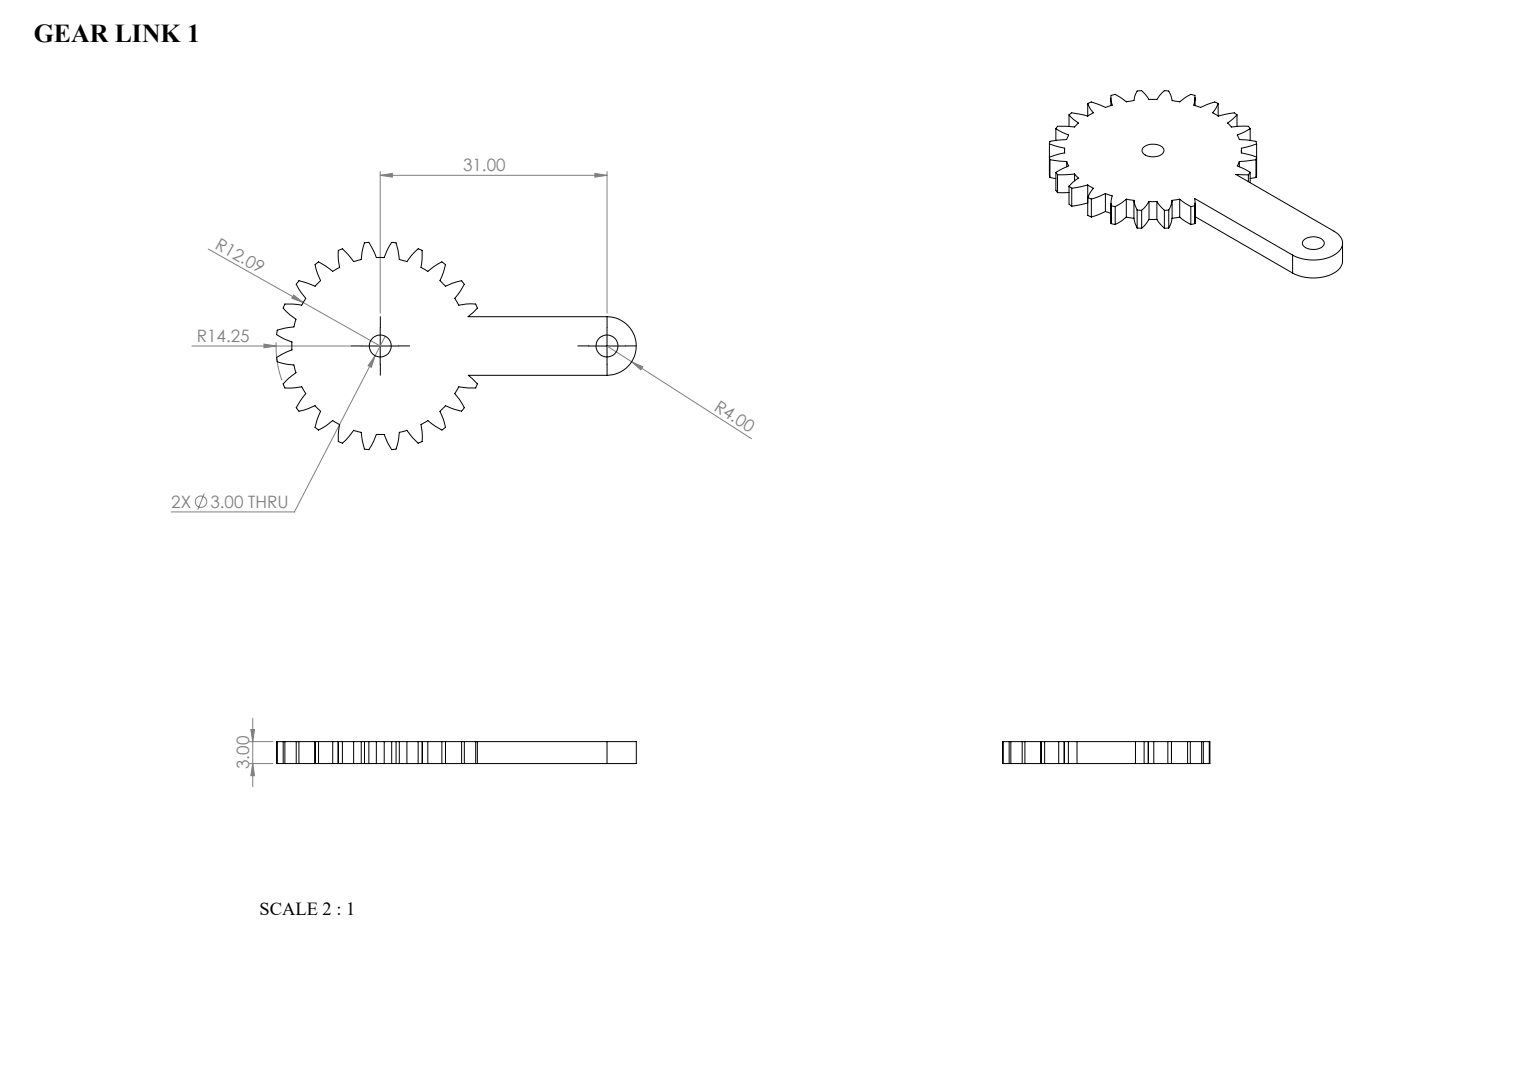
ISO-10303-21;
HEADER;
FILE_DESCRIPTION (('STEP AP214'),
    '1' );
FILE_NAME ('gear-link-1.step',
    '2026-10-11T23:18:24',
    ( '' ),
    ( '' ),
    'SwSTEP 2.0',
    'SolidWorks 2021',
    '' );
FILE_SCHEMA (( 'AUTOMOTIVE_DESIGN' ));
ENDSEC;

DATA;
#5=FACE_OUTER_BOUND ( 'NONE', #2599, .T. ) ;
#10=B_SPLINE_CURVE_WITH_KNOTS ( 'NONE', 3,
 ( #6640, #5405, #12919, #3466 ),
 .UNSPECIFIED., .F., .F.,
 ( 4, 4 ),
 ( 0.1547128134717859205, 1.000000000000000000 ),
 .UNSPECIFIED. ) ;
#12=DIRECTION ( 'NONE',  ( 0.000000000000000000, 0.000000000000000000, 1.000000000000000000 ) ) ;
#13=CARTESIAN_POINT ( 'NONE',  ( 0.000000000000000000, 3.000000000000000000, 0.000000000000000000 ) ) ;
#14=AXIS2_PLACEMENT_3D ( 'NONE', #3049, #7055, #9450 ) ;
#21=B_SPLINE_CURVE_WITH_KNOTS ( 'NONE', 3,
 ( #12632, #11655, #3183, #102 ),
 .UNSPECIFIED., .F., .F.,
 ( 4, 4 ),
 ( 0.1547128134717859205, 1.000000000000000000 ),
 .UNSPECIFIED. ) ;
#30=DIRECTION ( 'NONE',  ( -0.000000000000000000, -1.000000000000000000, -0.000000000000000000 ) ) ;
#35=DIRECTION ( 'NONE',  ( 0.000000000000000000, 1.000000000000000000, 0.000000000000000000 ) ) ;
#40=AXIS2_PLACEMENT_3D ( 'NONE', #1430, #2390, #10728 ) ;
#41=VECTOR ( 'NONE', #1784, 1000.000000000000000 ) ;
#55=CARTESIAN_POINT ( 'NONE',  ( -4.564691384634503635, 3.000000000000000000, 12.76342233970727769 ) ) ;
#57=ORIENTED_EDGE ( 'NONE', *, *, #11037, .F. ) ;
#59=ADVANCED_FACE ( 'NONE', ( #12400 ), #9143, .T. ) ;
#60=DIRECTION ( 'NONE',  ( -0.000000000000000000, -1.000000000000000000, -0.000000000000000000 ) ) ;
#61=EDGE_CURVE ( 'NONE', #8421, #357, #9412, .T. ) ;
#69=AXIS2_PLACEMENT_3D ( 'NONE', #2315, #6513, #10716 ) ;
#71=CARTESIAN_POINT ( 'NONE',  ( 2.161962830978782613, 0.000000000000000000, 14.08504230442586369 ) ) ;
#74=CARTESIAN_POINT ( 'NONE',  ( 5.170206418547656391, 3.000000000000000000, 13.27898586450067064 ) ) ;
#78=FACE_OUTER_BOUND ( 'NONE', #11147, .T. ) ;
#79=AXIS2_PLACEMENT_3D ( 'NONE', #10784, #8462, #2387 ) ;
#83=LINE ( 'NONE', #6330, #6796 ) ;
#90=CARTESIAN_POINT ( 'NONE',  ( 13.04554897075799502, 0.000000000000000000, 5.733772933379473358 ) ) ;
#91=LINE ( 'NONE', #6076, #1434 ) ;
#93=CIRCLE ( 'NONE', #9082, 12.08999999999737085 ) ;
#94=ORIENTED_EDGE ( 'NONE', *, *, #1256, .F. ) ;
#97=VERTEX_POINT ( 'NONE', #7219 ) ;
#99=CARTESIAN_POINT ( 'NONE',  ( 0.000000000000000000, 0.000000000000000000, 0.000000000000000000 ) ) ;
#102=CARTESIAN_POINT ( 'NONE',  ( -14.08504230442587790, 0.000000000000000000, -2.161962830978695571 ) ) ;
#106=CARTESIAN_POINT ( 'NONE',  ( 12.89546620003432764, 3.000000000000000000, -4.733530556166651415 ) ) ;
#109=CYLINDRICAL_SURFACE ( 'NONE', #708, 12.08999999999737440 ) ;
#110=CARTESIAN_POINT ( 'NONE',  ( -8.430890348300632553, 0.000000000000000000, -11.48836750521723538 ) ) ;
#112=EDGE_LOOP ( 'NONE', ( #12398, #1817, #7232, #6779 ) ) ;
#113=EDGE_CURVE ( 'NONE', #9400, #10019, #10289, .T. ) ;
#115=AXIS2_PLACEMENT_3D ( 'NONE', #683, #10945, #4876 ) ;
#116=VERTEX_POINT ( 'NONE', #11558 ) ;
#119=EDGE_LOOP ( 'NONE', ( #1078, #10235 ) ) ;
#128=LINE ( 'NONE', #8180, #4659 ) ;
#129=ORIENTED_EDGE ( 'NONE', *, *, #3513, .F. ) ;
#131=AXIS2_PLACEMENT_3D ( 'NONE', #780, #12143, #5869 ) ;
#139=DIRECTION ( 'NONE',  ( -0.000000000000000000, -1.000000000000000000, -0.000000000000000000 ) ) ;
#140=CARTESIAN_POINT ( 'NONE',  ( 12.03251085770905959, 3.000000000000000000, 3.999999998926332179 ) ) ;
#146=CARTESIAN_POINT ( 'NONE',  ( 12.03251085770905959, 0.000000000000000000, 3.999999998926332179 ) ) ;
#149=ORIENTED_EDGE ( 'NONE', *, *, #3145, .T. ) ;
#151=EDGE_CURVE ( 'NONE', #10361, #2347, #9475, .T. ) ;
#152=CARTESIAN_POINT ( 'NONE',  ( 4.564691384634508964, 3.000000000000000000, -12.76342233970727413 ) ) ;
#153=ADVANCED_FACE ( 'NONE', ( #4377 ), #6607, .F. ) ;
#158=ORIENTED_EDGE ( 'NONE', *, *, #6115, .F. ) ;
#159=CARTESIAN_POINT ( 'NONE',  ( -1.557181465540760534, 3.000000000000000000, -14.16466328168009703 ) ) ;
#163=ORIENTED_EDGE ( 'NONE', *, *, #6136, .T. ) ;
#164=DIRECTION ( 'NONE',  ( 0.000000000000000000, 0.000000000000000000, 1.000000000000000000 ) ) ;
#169=CARTESIAN_POINT ( 'NONE',  ( 2.604399508763944660, 3.000000000000000000, -11.80615107470197600 ) ) ;
#172=CARTESIAN_POINT ( 'NONE',  ( 12.46219022525837694, 3.000000000000000000, -4.344528055836598845 ) ) ;
#174=CYLINDRICAL_SURFACE ( 'NONE', #2308, 12.08999999999737440 ) ;
#177=B_SPLINE_SURFACE_WITH_KNOTS ( 'NONE', 3, 1, ( 
 ( #3234, #4074 ),
 ( #11315, #11514 ),
 ( #3171, #9382 ),
 ( #841, #13580 ) ),
 .UNSPECIFIED., .F., .F., .F.,
 ( 4, 4 ),
 ( 2, 2 ),
 ( 0.1547128134717859205, 1.000000000000000000 ),
 ( 0.000000000000000000, 1.000000000000000000 ),
 .UNSPECIFIED. ) ;
#179=ORIENTED_EDGE ( 'NONE', *, *, #10718, .F. ) ;
#185=CARTESIAN_POINT ( 'NONE',  ( 1.557181465540672161, 3.000000000000000000, -14.16466328168010591 ) ) ;
#186=DIRECTION ( 'NONE',  ( 0.000000000000000000, 1.000000000000000000, 0.000000000000000000 ) ) ;
#189=ORIENTED_EDGE ( 'NONE', *, *, #8491, .T. ) ;
#194=CARTESIAN_POINT ( 'NONE',  ( -8.158651161643904359, 3.000000000000000000, -8.922136023539605887 ) ) ;
#199=DIRECTION ( 'NONE',  ( -0.000000000000000000, -1.000000000000000000, -0.000000000000000000 ) ) ;
#203=DIRECTION ( 'NONE',  ( 0.000000000000000000, 0.000000000000000000, 1.000000000000000000 ) ) ;
#205=VERTEX_POINT ( 'NONE', #6448 ) ;
#206=ORIENTED_EDGE ( 'NONE', *, *, #10658, .F. ) ;
#216=CARTESIAN_POINT ( 'NONE',  ( -13.33579367773357482, 0.000000000000000000, 2.428572470324200427 ) ) ;
#230=AXIS2_PLACEMENT_3D ( 'NONE', #6911, #11119, #1688 ) ;
#233=CARTESIAN_POINT ( 'NONE',  ( 9.600126836553261711, 3.000000000000000000, 8.482622935103766082 ) ) ;
#239=AXIS2_PLACEMENT_3D ( 'NONE', #13533, #6287, #2844 ) ;
#244=VECTOR ( 'NONE', #1493, 1000.000000000000000 ) ;
#245=LINE ( 'NONE', #7737, #3762 ) ;
#246=CARTESIAN_POINT ( 'NONE',  ( 7.723663868796767140, 0.000000000000000000, 11.13895890373327191 ) ) ;
#251=ORIENTED_EDGE ( 'NONE', *, *, #1134, .T. ) ;
#260=DIRECTION ( 'NONE',  ( 0.000000000000000000, 1.000000000000000000, 0.000000000000000000 ) ) ;
#261=CIRCLE ( 'NONE', #2893, 12.08999999999737440 ) ;
#267=ORIENTED_EDGE ( 'NONE', *, *, #5862, .F. ) ;
#270=CARTESIAN_POINT ( 'NONE',  ( 0.5400000000008001733, 0.000000000000000000, 12.07793442604883616 ) ) ;
#277=CARTESIAN_POINT ( 'NONE',  ( 5.571313494980134173, 0.000000000000000000, -10.72979803820132005 ) ) ;
#284=VERTEX_POINT ( 'NONE', #2910 ) ;
#286=VECTOR ( 'NONE', #8892, 1000.000000000000000 ) ;
#294=CIRCLE ( 'NONE', #2053, 12.08999999999737263 ) ;
#299=B_SPLINE_CURVE_WITH_KNOTS ( 'NONE', 3,
 ( #9811, #1338, #2514, #4372 ),
 .UNSPECIFIED., .F., .F.,
 ( 4, 4 ),
 ( 0.1547128134717859205, 1.000000000000000000 ),
 .UNSPECIFIED. ) ;
#302=CARTESIAN_POINT ( 'NONE',  ( 10.33484986938308481, 3.000000000000000000, -8.771102293099065861 ) ) ;
#303=EDGE_CURVE ( 'NONE', #781, #13268, #10919, .T. ) ;
#307=CARTESIAN_POINT ( 'NONE',  ( -8.914835885878282795, 0.000000000000000000, -11.11702303352191556 ) ) ;
#309=CIRCLE ( 'NONE', #12190, 12.08999999999737263 ) ;
#310=EDGE_LOOP ( 'NONE', ( #4705, #3628, #1202, #9996 ) ) ;
#313=VERTEX_POINT ( 'NONE', #10072 ) ;
#320=DIRECTION ( 'NONE',  ( 0.000000000000000000, 1.000000000000000000, 0.000000000000000000 ) ) ;
#322=DIRECTION ( 'NONE',  ( -0.000000000000000000, -1.000000000000000000, -0.000000000000000000 ) ) ;
#324=ORIENTED_EDGE ( 'NONE', *, *, #508, .F. ) ;
#327=CIRCLE ( 'NONE', #13072, 14.25000000000000000 ) ;
#331=FACE_OUTER_BOUND ( 'NONE', #928, .T. ) ;
#333=CARTESIAN_POINT ( 'NONE',  ( 10.67828022838850366, 0.000000000000000000, -7.077546079049271022 ) ) ;
#334=VECTOR ( 'NONE', #12084, 1000.000000000000000 ) ;
#335=CARTESIAN_POINT ( 'NONE',  ( -8.914835885878215294, 0.000000000000000000, 11.11702303352197063 ) ) ;
#340=ORIENTED_EDGE ( 'NONE', *, *, #11404, .T. ) ;
#342=ORIENTED_EDGE ( 'NONE', *, *, #5264, .T. ) ;
#349=CARTESIAN_POINT ( 'NONE',  ( 5.733772933379474246, 3.000000000000000000, -13.04554897075799502 ) ) ;
#351=B_SPLINE_SURFACE_WITH_KNOTS ( 'NONE', 3, 1, ( 
 ( #13128, #5749 ),
 ( #9949, #12175 ),
 ( #2724, #6930 ),
 ( #3542, #2648 ) ),
 .UNSPECIFIED., .F., .F., .F.,
 ( 4, 4 ),
 ( 2, 2 ),
 ( 0.000000000000000000, 0.8452273900860258760 ),
 ( 0.000000000000000000, 1.000000000000000000 ),
 .UNSPECIFIED. ) ;
#353=EDGE_LOOP ( 'NONE', ( #2242, #11161, #428, #11636 ) ) ;
#355=DIRECTION ( 'NONE',  ( -0.000000000000000000, -1.000000000000000000, -0.000000000000000000 ) ) ;
#356=ORIENTED_EDGE ( 'NONE', *, *, #4337, .T. ) ;
#357=VERTEX_POINT ( 'NONE', #3539 ) ;
#364=EDGE_CURVE ( 'NONE', #8366, #10838, #2983, .T. ) ;
#367=ADVANCED_FACE ( 'NONE', ( #10218 ), #11113, .T. ) ;
#370=CARTESIAN_POINT ( 'NONE',  ( 11.11702303352194043, 3.000000000000000000, -8.914835885878249044 ) ) ;
#379=FACE_OUTER_BOUND ( 'NONE', #4363, .T. ) ;
#387=B_SPLINE_SURFACE_WITH_KNOTS ( 'NONE', 3, 1, ( 
 ( #6060, #3979 ),
 ( #1786, #3020 ),
 ( #2059, #9286 ),
 ( #760, #7090 ) ),
 .UNSPECIFIED., .F., .F., .F.,
 ( 4, 4 ),
 ( 2, 2 ),
 ( 0.000000000000000000, 0.8452273900860258760 ),
 ( 0.000000000000000000, 1.000000000000000000 ),
 .UNSPECIFIED. ) ;
#389=ORIENTED_EDGE ( 'NONE', *, *, #7985, .T. ) ;
#393=CARTESIAN_POINT ( 'NONE',  ( -12.78643498603817896, 0.000000000000000000, 0.7901945867173603144 ) ) ;
#394=LINE ( 'NONE', #9622, #244 ) ;
#397=CARTESIAN_POINT ( 'NONE',  ( -4.564691384634503635, 0.000000000000000000, 12.76342233970727769 ) ) ;
#399=ORIENTED_EDGE ( 'NONE', *, *, #5721, .T. ) ;
#401=ORIENTED_EDGE ( 'NONE', *, *, #13079, .T. ) ;
#403=ORIENTED_EDGE ( 'NONE', *, *, #2950, .F. ) ;
#408=CARTESIAN_POINT ( 'NONE',  ( 8.760376775873721655, 3.000000000000000000, -10.34346111134700585 ) ) ;
#409=FACE_OUTER_BOUND ( 'NONE', #1971, .T. ) ;
#410=ORIENTED_EDGE ( 'NONE', *, *, #2346, .T. ) ;
#414=ORIENTED_EDGE ( 'NONE', *, *, #8684, .F. ) ;
#416=ORIENTED_EDGE ( 'NONE', *, *, #2484, .T. ) ;
#428=ORIENTED_EDGE ( 'NONE', *, *, #6747, .F. ) ;
#433=ADVANCED_FACE ( 'NONE', ( #4281 ), #6408, .T. ) ;
#436=CARTESIAN_POINT ( 'NONE',  ( 31.00000000000000000, 3.000000000000000000, 3.999999998926329514 ) ) ;
#442=DIRECTION ( 'NONE',  ( -0.000000000000000000, -1.000000000000000000, -0.000000000000000000 ) ) ;
#443=AXIS2_PLACEMENT_3D ( 'NONE', #4842, #10911, #11044 ) ;
#453=VECTOR ( 'NONE', #9150, 1000.000000000000000 ) ;
#459=FACE_OUTER_BOUND ( 'NONE', #9234, .T. ) ;
#466=ORIENTED_EDGE ( 'NONE', *, *, #3127, .F. ) ;
#475=CARTESIAN_POINT ( 'NONE',  ( 0.000000000000000000, 3.000000000000000000, 0.000000000000000000 ) ) ;
#478=CARTESIAN_POINT ( 'NONE',  ( 0.000000000000000000, 3.000000000000000000, 0.000000000000000000 ) ) ;
#482=EDGE_LOOP ( 'NONE', ( #4350, #4366, #12937, #9187 ) ) ;
#484=CIRCLE ( 'NONE', #8176, 12.08999999999737440 ) ;
#487=DIRECTION ( 'NONE',  ( -0.000000000000000000, -1.000000000000000000, -0.000000000000000000 ) ) ;
#495=CARTESIAN_POINT ( 'NONE',  ( -12.25836857253663759, 0.000000000000000000, -5.784789447945487773 ) ) ;
#496=CARTESIAN_POINT ( 'NONE',  ( 13.27898586450067242, 0.000000000000000000, -5.170206418547655502 ) ) ;
#500=VERTEX_POINT ( 'NONE', #11383 ) ;
#508=EDGE_CURVE ( 'NONE', #12112, #12067, #13480, .T. ) ;
#509=CARTESIAN_POINT ( 'NONE',  ( -13.33579367773357482, 0.000000000000000000, 2.428572470324200427 ) ) ;
#523=VERTEX_POINT ( 'NONE', #12504 ) ;
#525=VERTEX_POINT ( 'NONE', #8535 ) ;
#527=VECTOR ( 'NONE', #5207, 1000.000000000000000 ) ;
#531=EDGE_CURVE ( 'NONE', #8124, #10022, #4668, .T. ) ;
#543=ORIENTED_EDGE ( 'NONE', *, *, #11120, .F. ) ;
#544=VERTEX_POINT ( 'NONE', #6210 ) ;
#545=CARTESIAN_POINT ( 'NONE',  ( -2.604399508763951321, 3.000000000000000000, 11.80615107470197422 ) ) ;
#546=ORIENTED_EDGE ( 'NONE', *, *, #12833, .F. ) ;
#547=CARTESIAN_POINT ( 'NONE',  ( 0.000000000000000000, 3.000000000000000000, 0.000000000000000000 ) ) ;
#550=CIRCLE ( 'NONE', #6708, 12.08999999999737618 ) ;
#555=DIRECTION ( 'NONE',  ( 0.000000000000000000, 0.000000000000000000, -1.000000000000000000 ) ) ;
#561=EDGE_LOOP ( 'NONE', ( #2555, #11444 ) ) ;
#562=AXIS2_PLACEMENT_3D ( 'NONE', #11848, #2406, #1375 ) ;
#566=ORIENTED_EDGE ( 'NONE', *, *, #7660, .T. ) ;
#571=CARTESIAN_POINT ( 'NONE',  ( 1.557181465540758758, 3.000000000000000000, 14.16466328168009881 ) ) ;
#575=ORIENTED_EDGE ( 'NONE', *, *, #6812, .F. ) ;
#579=B_SPLINE_SURFACE_WITH_KNOTS ( 'NONE', 3, 1, ( 
 ( #4760, #8946 ),
 ( #13160, #3708 ),
 ( #6886, #7909 ),
 ( #10120, #3025 ) ),
 .UNSPECIFIED., .F., .F., .F.,
 ( 4, 4 ),
 ( 2, 2 ),
 ( 0.000000000000000000, 0.8452273900860258760 ),
 ( 0.000000000000000000, 1.000000000000000000 ),
 .UNSPECIFIED. ) ;
#582=B_SPLINE_CURVE_WITH_KNOTS ( 'NONE', 3,
 ( #1871, #5783, #10055, #4884 ),
 .UNSPECIFIED., .F., .F.,
 ( 4, 4 ),
 ( 0.000000000000000000, 0.8452273900860258760 ),
 .UNSPECIFIED. ) ;
#597=VERTEX_POINT ( 'NONE', #11720 ) ;
#602=DIRECTION ( 'NONE',  ( -0.000000000000000000, -1.000000000000000000, -0.000000000000000000 ) ) ;
#605=CARTESIAN_POINT ( 'NONE',  ( -3.647470871583628593, 0.000000000000000000, 11.52666717836884125 ) ) ;
#611=DIRECTION ( 'NONE',  ( -0.000000000000000000, -1.000000000000000000, -0.000000000000000000 ) ) ;
#612=ORIENTED_EDGE ( 'NONE', *, *, #3358, .T. ) ;
#617=CARTESIAN_POINT ( 'NONE',  ( 0.000000000000000000, 0.000000000000000000, -1.500000000000000222 ) ) ;
#619=CARTESIAN_POINT ( 'NONE',  ( -6.506507307819711095, 0.000000000000000000, 10.18987059060247624 ) ) ;
#620=CARTESIAN_POINT ( 'NONE',  ( 8.922226997226882617, 3.000000000000000000, 8.158551673544282679 ) ) ;
#625=ORIENTED_EDGE ( 'NONE', *, *, #2071, .F. ) ;
#627=CARTESIAN_POINT ( 'NONE',  ( -1.557181465540221188, 3.000000000000000000, 14.16466328168015743 ) ) ;
#638=CARTESIAN_POINT ( 'NONE',  ( -5.784789447945489549, 3.000000000000000000, 12.25836857253663581 ) ) ;
#643=DIRECTION ( 'NONE',  ( 0.000000000000000000, 0.000000000000000000, -1.000000000000000000 ) ) ;
#651=CARTESIAN_POINT ( 'NONE',  ( -7.723663868796776910, 3.000000000000000000, -11.13895890373326303 ) ) ;
#652=CARTESIAN_POINT ( 'NONE',  ( 2.604399508763944660, 3.000000000000000000, -11.80615107470197600 ) ) ;
#653=CARTESIAN_POINT ( 'NONE',  ( -5.170206418547658167, 0.000000000000000000, -13.27898586450066887 ) ) ;
#654=CARTESIAN_POINT ( 'NONE',  ( -3.647599401157691545, 3.000000000000000000, -11.52662650599084238 ) ) ;
#655=VERTEX_POINT ( 'NONE', #11922 ) ;
#656=ORIENTED_EDGE ( 'NONE', *, *, #9257, .F. ) ;
#659=CARTESIAN_POINT ( 'NONE',  ( -8.158551673544284455, 3.000000000000000000, 8.922226997226891498 ) ) ;
#668=DIRECTION ( 'NONE',  ( 0.000000000000000000, 0.000000000000000000, -1.000000000000000000 ) ) ;
#669=CARTESIAN_POINT ( 'NONE',  ( -4.056222772158361245, 0.000000000000000000, 12.16218796965919324 ) ) ;
#673=CARTESIAN_POINT ( 'NONE',  ( -2.414978278956346092, 0.000000000000000000, 13.33788847341978467 ) ) ;
#680=CARTESIAN_POINT ( 'NONE',  ( 6.506507307819716424, 3.000000000000000000, -10.18987059060247269 ) ) ;
#682=CIRCLE ( 'NONE', #5520, 12.08999999999737440 ) ;
#683=CARTESIAN_POINT ( 'NONE',  ( 0.000000000000000000, 0.000000000000000000, 0.000000000000000000 ) ) ;
#684=CIRCLE ( 'NONE', #8370, 12.08999999999737263 ) ;
#686=AXIS2_PLACEMENT_3D ( 'NONE', #5417, #1154, #13562 ) ;
#688=VERTEX_POINT ( 'NONE', #10752 ) ;
#689=CARTESIAN_POINT ( 'NONE',  ( 0.000000000000000000, 3.000000000000000000, 0.000000000000000000 ) ) ;
#690=EDGE_CURVE ( 'NONE', #9707, #1933, #9292, .T. ) ;
#708=AXIS2_PLACEMENT_3D ( 'NONE', #11662, #2221, #6424 ) ;
#709=ORIENTED_EDGE ( 'NONE', *, *, #2346, .F. ) ;
#714=CARTESIAN_POINT ( 'NONE',  ( 8.771102293099069414, 0.000000000000000000, 10.33484986938308303 ) ) ;
#719=CARTESIAN_POINT ( 'NONE',  ( -13.04554897075796127, 0.000000000000000000, 5.733772933379547077 ) ) ;
#733=ORIENTED_EDGE ( 'NONE', *, *, #13367, .T. ) ;
#734=DIRECTION ( 'NONE',  ( -0.000000000000000000, -1.000000000000000000, -0.000000000000000000 ) ) ;
#738=CIRCLE ( 'NONE', #1389, 12.08999999999737440 ) ;
#744=CARTESIAN_POINT ( 'NONE',  ( -13.50994833511691340, 0.000000000000000000, -1.105736515254444052 ) ) ;
#750=CARTESIAN_POINT ( 'NONE',  ( -13.04554897075795949, 3.000000000000000000, 5.733772933379550629 ) ) ;
#751=CIRCLE ( 'NONE', #6016, 12.08999999999737440 ) ;
#753=EDGE_CURVE ( 'NONE', #11680, #11839, #5026, .T. ) ;
#755=CARTESIAN_POINT ( 'NONE',  ( 11.11702303352194043, 0.000000000000000000, -8.914835885878249044 ) ) ;
#760=CARTESIAN_POINT ( 'NONE',  ( -8.922136023539609440, 3.000000000000000000, 8.158651161643900807 ) ) ;
#769=FACE_OUTER_BOUND ( 'NONE', #7814, .T. ) ;
#773=AXIS2_PLACEMENT_3D ( 'NONE', #5480, #10594, #1085 ) ;
#774=ORIENTED_EDGE ( 'NONE', *, *, #4675, .F. ) ;
#775=DIRECTION ( 'NONE',  ( -0.000000000000000000, -1.000000000000000000, -0.000000000000000000 ) ) ;
#780=CARTESIAN_POINT ( 'NONE',  ( 0.000000000000000000, 0.000000000000000000, 0.000000000000000000 ) ) ;
#781=VERTEX_POINT ( 'NONE', #627 ) ;
#783=CARTESIAN_POINT ( 'NONE',  ( -14.16466328168009881, 3.000000000000000000, 1.557181465540760534 ) ) ;
#785=ORIENTED_EDGE ( 'NONE', *, *, #3659, .F. ) ;
#787=CARTESIAN_POINT ( 'NONE',  ( 0.000000000000000000, 3.000000000000000000, 0.000000000000000000 ) ) ;
#788=EDGE_CURVE ( 'NONE', #1247, #10439, #582, .T. ) ;
#796=CARTESIAN_POINT ( 'NONE',  ( -12.56087513340552242, 0.000000000000000000, 2.568302020731519253 ) ) ;
#797=DIRECTION ( 'NONE',  ( 0.000000000000000000, 0.000000000000000000, 1.000000000000000000 ) ) ;
#798=CARTESIAN_POINT ( 'NONE',  ( -13.50845331674225847, 3.000000000000000000, 1.119409668803372115 ) ) ;
#800=CARTESIAN_POINT ( 'NONE',  ( -6.506620931068715308, 3.000000000000000000, -10.18979803820051799 ) ) ;
#803=LINE ( 'NONE', #12094, #13042 ) ;
#806=ORIENTED_EDGE ( 'NONE', *, *, #6747, .T. ) ;
#807=ORIENTED_EDGE ( 'NONE', *, *, #13420, .F. ) ;
#817=CARTESIAN_POINT ( 'NONE',  ( -10.69794375946289655, 3.000000000000000000, -7.065816209474156118 ) ) ;
#818=CARTESIAN_POINT ( 'NONE',  ( 0.000000000000000000, 3.000000000000000000, -12.08999999999737440 ) ) ;
#820=B_SPLINE_CURVE_WITH_KNOTS ( 'NONE', 3,
 ( #13008, #12943, #6736, #7833 ),
 .UNSPECIFIED., .F., .F.,
 ( 4, 4 ),
 ( 0.1547128134717859205, 1.000000000000000000 ),
 .UNSPECIFIED. ) ;
#821=FACE_OUTER_BOUND ( 'NONE', #2364, .T. ) ;
#823=CARTESIAN_POINT ( 'NONE',  ( 0.7702044561450380744, 0.000000000000000000, -12.79759916868914615 ) ) ;
#824=DIRECTION ( 'NONE',  ( 0.000000000000000000, 0.000000000000000000, 1.000000000000000000 ) ) ;
#825=CARTESIAN_POINT ( 'NONE',  ( 5.731782959214990036, 0.000000000000000000, 11.46814821560793618 ) ) ;
#829=CARTESIAN_POINT ( 'NONE',  ( -12.76342233970728124, 3.000000000000000000, -4.564691384634500970 ) ) ;
#831=ORIENTED_EDGE ( 'NONE', *, *, #531, .F. ) ;
#839=DIRECTION ( 'NONE',  ( 0.000000000000000000, 0.000000000000000000, -1.000000000000000000 ) ) ;
#841=CARTESIAN_POINT ( 'NONE',  ( -13.04554897075799680, 3.000000000000000000, -5.733772933379471581 ) ) ;
#843=VERTEX_POINT ( 'NONE', #3647 ) ;
#846=VERTEX_POINT ( 'NONE', #2681 ) ;
#849=ORIENTED_EDGE ( 'NONE', *, *, #6154, .F. ) ;
#859=DIRECTION ( 'NONE',  ( -0.000000000000000000, -1.000000000000000000, -0.000000000000000000 ) ) ;
#862=DIRECTION ( 'NONE',  ( -0.000000000000000000, -1.000000000000000000, -0.000000000000000000 ) ) ;
#873=DIRECTION ( 'NONE',  ( -0.000000000000000000, -1.000000000000000000, -0.000000000000000000 ) ) ;
#874=CARTESIAN_POINT ( 'NONE',  ( 7.712570079660896916, 3.000000000000000000, -11.14709020439929432 ) ) ;
#875=DIRECTION ( 'NONE',  ( -0.000000000000000000, -1.000000000000000000, -0.000000000000000000 ) ) ;
#878=ADVANCED_FACE ( 'NONE', ( #769 ), #579, .F. ) ;
#880=CARTESIAN_POINT ( 'NONE',  ( 13.04554897075799502, 3.000000000000000000, 5.733772933379473358 ) ) ;
#883=DIRECTION ( 'NONE',  ( 0.000000000000000000, 1.000000000000000000, 0.000000000000000000 ) ) ;
#884=PRODUCT_CONTEXT ( 'NONE', #2816, 'mechanical' ) ;
#886=CARTESIAN_POINT ( 'NONE',  ( 5.571433138827823761, 3.000000000000000000, 10.72973591378220704 ) ) ;
#887=CARTESIAN_POINT ( 'NONE',  ( -11.48836750521723893, 3.000000000000000000, 8.430890348300625448 ) ) ;
#911=VERTEX_POINT ( 'NONE', #7174 ) ;
#917=ADVANCED_FACE ( 'NONE', ( #5 ), #1999, .T. ) ;
#921=CARTESIAN_POINT ( 'NONE',  ( 31.00000000000000000, 3.000000000000000000, -1.073670993220974656E-09 ) ) ;
#927=CARTESIAN_POINT ( 'NONE',  ( -2.568302020731516588, 0.000000000000000000, -12.56087513340552242 ) ) ;
#928=EDGE_LOOP ( 'NONE', ( #5189, #8417, #11342, #4818 ) ) ;
#931=B_SPLINE_CURVE_WITH_KNOTS ( 'NONE', 3,
 ( #11785, #6404, #10616, #7446 ),
 .UNSPECIFIED., .F., .F.,
 ( 4, 4 ),
 ( 0.000000000000000000, 0.8452273900860258760 ),
 .UNSPECIFIED. ) ;
#939=CYLINDRICAL_SURFACE ( 'NONE', #12631, 14.25000000000000178 ) ;
#946=EDGE_LOOP ( 'NONE', ( #12130, #12248, #7141, #189 ) ) ;
#947=ORIENTED_EDGE ( 'NONE', *, *, #12559, .T. ) ;
#948=CARTESIAN_POINT ( 'NONE',  ( 11.46847481510586775, 3.000000000000000000, 5.708888906988908829 ) ) ;
#951=CARTESIAN_POINT ( 'NONE',  ( 8.482622935103764306, 0.000000000000000000, -9.600126836553261711 ) ) ;
#957=ADVANCED_FACE ( 'NONE', ( #78 ), #10534, .T. ) ;
#958=CARTESIAN_POINT ( 'NONE',  ( 0.5398653231797245766, 0.000000000000000000, -12.07794044664754018 ) ) ;
#959=CARTESIAN_POINT ( 'NONE',  ( 12.48034623170854474, 3.000000000000000000, 4.337627373772809491 ) ) ;
#963=CARTESIAN_POINT ( 'NONE',  ( 12.03251085770905959, 0.000000000000000000, 3.999999998926332179 ) ) ;
#964=VECTOR ( 'NONE', #3111, 1000.000000000000000 ) ;
#972=VECTOR ( 'NONE', #2138, 1000.000000000000000 ) ;
#979=CARTESIAN_POINT ( 'NONE',  ( -5.571433138827826426, 3.000000000000000000, -10.72973591378220526 ) ) ;
#980=ORIENTED_EDGE ( 'NONE', *, *, #10718, .T. ) ;
#982=ORIENTED_EDGE ( 'NONE', *, *, #13564, .F. ) ;
#985=B_SPLINE_CURVE_WITH_KNOTS ( 'NONE', 3,
 ( #4368, #8556, #9667, #12778 ),
 .UNSPECIFIED., .F., .F.,
 ( 4, 4 ),
 ( 0.000000000000000000, 0.8452273900860258760 ),
 .UNSPECIFIED. ) ;
#986=EDGE_CURVE ( 'NONE', #1347, #525, #738, .T. ) ;
#987=EDGE_CURVE ( 'NONE', #13268, #8754, #11578, .T. ) ;
#988=ORIENTED_EDGE ( 'NONE', *, *, #11808, .T. ) ;
#993=B_SPLINE_CURVE_WITH_KNOTS ( 'NONE', 3,
 ( #11149, #12478, #3016, #10103 ),
 .UNSPECIFIED., .F., .F.,
 ( 4, 4 ),
 ( 0.1547128134717859205, 1.000000000000000000 ),
 .UNSPECIFIED. ) ;
#1000=CARTESIAN_POINT ( 'NONE',  ( 11.48836750521724070, 0.000000000000000000, 8.430890348300627224 ) ) ;
#1009=CARTESIAN_POINT ( 'NONE',  ( -8.914835885878282795, 3.000000000000000000, -11.11702303352191556 ) ) ;
#1011=DIRECTION ( 'NONE',  ( 0.000000000000000000, 0.000000000000000000, 1.000000000000000000 ) ) ;
#1013=CARTESIAN_POINT ( 'NONE',  ( -7.712570079660889810, 3.000000000000000000, 11.14709020439930320 ) ) ;
#1017=CARTESIAN_POINT ( 'NONE',  ( -11.48836750521728689, 3.000000000000000000, -8.430890348300561499 ) ) ;
#1021=CARTESIAN_POINT ( 'NONE',  ( -11.48836750521728867, 3.000000000000000000, -8.430890348300557946 ) ) ;
#1028=LINE ( 'NONE', #10468, #1408 ) ;
#1043=DIRECTION ( 'NONE',  ( -0.000000000000000000, -1.000000000000000000, -0.000000000000000000 ) ) ;
#1045=CARTESIAN_POINT ( 'NONE',  ( 0.000000000000000000, 0.000000000000000000, 0.000000000000000000 ) ) ;
#1046=EDGE_LOOP ( 'NONE', ( #8671, #13240, #543, #1474 ) ) ;
#1054=CARTESIAN_POINT ( 'NONE',  ( 0.000000000000000000, 3.000000000000000000, 0.000000000000000000 ) ) ;
#1055=DIRECTION ( 'NONE',  ( 0.000000000000000000, 0.000000000000000000, 1.000000000000000000 ) ) ;
#1058=DIRECTION ( 'NONE',  ( 0.000000000000000000, 0.000000000000000000, -1.000000000000000000 ) ) ;
#1061=VERTEX_POINT ( 'NONE', #7768 ) ;
#1063=VERTEX_POINT ( 'NONE', #2537 ) ;
#1065=ORIENTED_EDGE ( 'NONE', *, *, #6952, .T. ) ;
#1067=ORIENTED_EDGE ( 'NONE', *, *, #1799, .F. ) ;
#1072=CARTESIAN_POINT ( 'NONE',  ( 11.48836750521724070, 3.000000000000000000, 8.430890348300627224 ) ) ;
#1073=CARTESIAN_POINT ( 'NONE',  ( -6.506507307819711095, 3.000000000000000000, 10.18987059060247624 ) ) ;
#1078=ORIENTED_EDGE ( 'NONE', *, *, #6023, .T. ) ;
#1085=DIRECTION ( 'NONE',  ( 0.000000000000000000, 0.000000000000000000, 1.000000000000000000 ) ) ;
#1089=B_SPLINE_CURVE_WITH_KNOTS ( 'NONE', 3,
 ( #12109, #4593, #4863, #1710 ),
 .UNSPECIFIED., .F., .F.,
 ( 4, 4 ),
 ( 0.000000000000000000, 0.8452273900860258760 ),
 .UNSPECIFIED. ) ;
#1090=VERTEX_POINT ( 'NONE', #6467 ) ;
#1091=VERTEX_POINT ( 'NONE', #9764 ) ;
#1098=( NAMED_UNIT ( * ) SI_UNIT ( $, .STERADIAN. ) SOLID_ANGLE_UNIT ( ) );
#1101=CARTESIAN_POINT ( 'NONE',  ( -10.67828022838850721, 3.000000000000000000, 7.077546079049267469 ) ) ;
#1103=VECTOR ( 'NONE', #6151, 1000.000000000000000 ) ;
#1104=CARTESIAN_POINT ( 'NONE',  ( -14.08504230442586369, 0.000000000000000000, 2.161962830978781724 ) ) ;
#1109=ORIENTED_EDGE ( 'NONE', *, *, #8696, .F. ) ;
#1111=VERTEX_POINT ( 'NONE', #2338 ) ;
#1112=CARTESIAN_POINT ( 'NONE',  ( -8.914835885878282795, 0.000000000000000000, -11.11702303352191556 ) ) ;
#1114=AXIS2_PLACEMENT_3D ( 'NONE', #5964, #10032, #10093 ) ;
#1118=DIRECTION ( 'NONE',  ( -0.000000000000000000, -1.000000000000000000, -0.000000000000000000 ) ) ;
#1120=DIRECTION ( 'NONE',  ( 0.000000000000000000, 1.000000000000000000, 0.000000000000000000 ) ) ;
#1126=CARTESIAN_POINT ( 'NONE',  ( 0.000000000000000000, 3.000000000000000000, -1.500000000000000222 ) ) ;
#1128=CARTESIAN_POINT ( 'NONE',  ( 3.647599401157688437, 0.000000000000000000, 11.52662650599083882 ) ) ;
#1133=EDGE_LOOP ( 'NONE', ( #9505, #3278, #13431, #10279 ) ) ;
#1134=EDGE_CURVE ( 'NONE', #7270, #9350, #11725, .T. ) ;
#1139=FACE_OUTER_BOUND ( 'NONE', #4650, .T. ) ;
#1142=VERTEX_POINT ( 'NONE', #10736 ) ;
#1144=ORIENTED_EDGE ( 'NONE', *, *, #7271, .F. ) ;
#1148=EDGE_CURVE ( 'NONE', #8355, #2851, #12877, .T. ) ;
#1154=DIRECTION ( 'NONE',  ( 0.000000000000000000, 1.000000000000000000, 0.000000000000000000 ) ) ;
#1156=CARTESIAN_POINT ( 'NONE',  ( -12.25836857253663759, 3.000000000000000000, -5.784789447945487773 ) ) ;
#1158=DIRECTION ( 'NONE',  ( -0.000000000000000000, -1.000000000000000000, -0.000000000000000000 ) ) ;
#1162=VERTEX_POINT ( 'NONE', #13006 ) ;
#1165=MECHANICAL_DESIGN_GEOMETRIC_PRESENTATION_REPRESENTATION('',(#11512),#8633);
#1169=FACE_OUTER_BOUND ( 'NONE', #1046, .T. ) ;
#1170=B_SPLINE_CURVE_WITH_KNOTS ( 'NONE', 3,
 ( #10667, #12996, #2455, #1227 ),
 .UNSPECIFIED., .F., .F.,
 ( 4, 4 ),
 ( 0.1547128134717859205, 1.000000000000000000 ),
 .UNSPECIFIED. ) ;
#1175=CIRCLE ( 'NONE', #6230, 14.25000000000000178 ) ;
#1178=DIRECTION ( 'NONE',  ( 0.000000000000000000, 0.000000000000000000, -1.000000000000000000 ) ) ;
#1179=EDGE_LOOP ( 'NONE', ( #9943, #1067, #11868, #4169 ) ) ;
#1180=DIRECTION ( 'NONE',  ( 0.000000000000000000, 0.000000000000000000, -1.000000000000000000 ) ) ;
#1183=EDGE_CURVE ( 'NONE', #6311, #7408, #12402, .T. ) ;
#1186=CARTESIAN_POINT ( 'NONE',  ( 0.000000000000000000, 3.000000000000000000, 0.000000000000000000 ) ) ;
#1193=CARTESIAN_POINT ( 'NONE',  ( -12.16218796965919324, 3.000000000000000000, -4.056222772158363021 ) ) ;
#1196=CARTESIAN_POINT ( 'NONE',  ( 11.14709020439929787, 0.000000000000000000, 7.712570079660892475 ) ) ;
#1201=EDGE_CURVE ( 'NONE', #9963, #12046, #1703, .T. ) ;
#1202=ORIENTED_EDGE ( 'NONE', *, *, #10865, .F. ) ;
#1203=EDGE_CURVE ( 'NONE', #4274, #6311, #9519, .T. ) ;
#1207=EDGE_CURVE ( 'NONE', #8335, #9473, #5903, .T. ) ;
#1213=DIRECTION ( 'NONE',  ( 0.000000000000000000, 1.000000000000000000, 0.000000000000000000 ) ) ;
#1215=CARTESIAN_POINT ( 'NONE',  ( -14.16466328168010769, 0.000000000000000000, -1.557181465540673271 ) ) ;
#1227=CARTESIAN_POINT ( 'NONE',  ( -1.557181465540760534, 3.000000000000000000, -14.16466328168009703 ) ) ;
#1230=CARTESIAN_POINT ( 'NONE',  ( -5.733772933379540859, 3.000000000000000000, -13.04554897075796660 ) ) ;
#1235=VERTEX_POINT ( 'NONE', #750 ) ;
#1236=DIRECTION ( 'NONE',  ( 0.000000000000000000, 0.000000000000000000, 1.000000000000000000 ) ) ;
#1240=CARTESIAN_POINT ( 'NONE',  ( 0.000000000000000000, 3.000000000000000000, 0.000000000000000000 ) ) ;
#1246=CARTESIAN_POINT ( 'NONE',  ( -11.52666717836884125, 0.000000000000000000, -3.647470871583627705 ) ) ;
#1247=VERTEX_POINT ( 'NONE', #4666 ) ;
#1252=CARTESIAN_POINT ( 'NONE',  ( 0.000000000000000000, 3.000000000000000000, 0.000000000000000000 ) ) ;
#1256=EDGE_CURVE ( 'NONE', #500, #284, #294, .T. ) ;
#1259=CARTESIAN_POINT ( 'NONE',  ( 11.11702303352196708, 3.000000000000000000, 8.914835885878218846 ) ) ;
#1261=ORIENTED_EDGE ( 'NONE', *, *, #5620, .F. ) ;
#1262=DIRECTION ( 'NONE',  ( 0.000000000000000000, 1.000000000000000000, 0.000000000000000000 ) ) ;
#1270=EDGE_CURVE ( 'NONE', #9400, #12697, #9064, .T. ) ;
#1274=EDGE_CURVE ( 'NONE', #9473, #11839, #12226, .T. ) ;
#1275=CYLINDRICAL_SURFACE ( 'NONE', #5106, 14.24999999999999822 ) ;
#1293=ORIENTED_EDGE ( 'NONE', *, *, #3145, .F. ) ;
#1298=ADVANCED_FACE ( 'NONE', ( #5763 ), #9413, .T. ) ;
#1299=CARTESIAN_POINT ( 'NONE',  ( 10.69794375946289655, 3.000000000000000000, 7.065816209474157006 ) ) ;
#1302=DIRECTION ( 'NONE',  ( 0.000000000000000000, 0.000000000000000000, 1.000000000000000000 ) ) ;
#1306=EDGE_LOOP ( 'NONE', ( #12592, #5558, #11855, #389 ) ) ;
#1307=LINE ( 'NONE', #11714, #1392 ) ;
#1312=DIRECTION ( 'NONE',  ( 0.000000000000000000, 1.000000000000000000, 0.000000000000000000 ) ) ;
#1327=ORIENTED_EDGE ( 'NONE', *, *, #8998, .F. ) ;
#1331=CARTESIAN_POINT ( 'NONE',  ( 0.000000000000000000, 3.000000000000000000, 0.000000000000000000 ) ) ;
#1333=DIRECTION ( 'NONE',  ( -0.000000000000000000, -1.000000000000000000, -0.000000000000000000 ) ) ;
#1338=CARTESIAN_POINT ( 'NONE',  ( -2.546103534247749600, 3.000000000000000000, 12.55526518755974585 ) ) ;
#1347=VERTEX_POINT ( 'NONE', #818 ) ;
#1357=CARTESIAN_POINT ( 'NONE',  ( 4.577511697546072789, 3.000000000000000000, 12.75843939030335505 ) ) ;
#1360=EDGE_LOOP ( 'NONE', ( #2486, #7663, #2721, #8694 ) ) ;
#1365=ADVANCED_FACE ( 'NONE', ( #12532 ), #1682, .F. ) ;
#1371=CARTESIAN_POINT ( 'NONE',  ( -5.733772933379540859, 3.000000000000000000, -13.04554897075796660 ) ) ;
#1372=DIRECTION ( 'NONE',  ( -0.000000000000000000, -1.000000000000000000, -0.000000000000000000 ) ) ;
#1375=DIRECTION ( 'NONE',  ( 0.000000000000000000, 0.000000000000000000, -1.000000000000000000 ) ) ;
#1389=AXIS2_PLACEMENT_3D ( 'NONE', #12610, #3225, #12545 ) ;
#1392=VECTOR ( 'NONE', #4408, 1000.000000000000000 ) ;
#1396=DIRECTION ( 'NONE',  ( -0.000000000000000000, -1.000000000000000000, -0.000000000000000000 ) ) ;
#1406=VERTEX_POINT ( 'NONE', #11126 ) ;
#1408=VECTOR ( 'NONE', #8380, 1000.000000000000000 ) ;
#1412=CIRCLE ( 'NONE', #7350, 12.08999999999737618 ) ;
#1417=CARTESIAN_POINT ( 'NONE',  ( -14.08504230442587790, 3.000000000000000000, -2.161962830978695571 ) ) ;
#1420=ORIENTED_EDGE ( 'NONE', *, *, #753, .T. ) ;
#1424=VECTOR ( 'NONE', #487, 1000.000000000000000 ) ;
#1427=CARTESIAN_POINT ( 'NONE',  ( 8.430890348300625448, 0.000000000000000000, 11.48836750521723893 ) ) ;
#1430=CARTESIAN_POINT ( 'NONE',  ( 0.000000000000000000, 0.000000000000000000, 0.000000000000000000 ) ) ;
#1434=VECTOR ( 'NONE', #1043, 1000.000000000000000 ) ;
#1437=VERTEX_POINT ( 'NONE', #653 ) ;
#1449=CARTESIAN_POINT ( 'NONE',  ( 8.158551673544288008, 0.000000000000000000, -8.922226997226886169 ) ) ;
#1451=ORIENTED_EDGE ( 'NONE', *, *, #8998, .T. ) ;
#1453=EDGE_CURVE ( 'NONE', #3691, #11432, #13398, .T. ) ;
#1455=EDGE_CURVE ( 'NONE', #3087, #8384, #6921, .T. ) ;
#1460=ORIENTED_EDGE ( 'NONE', *, *, #6068, .F. ) ;
#1464=CARTESIAN_POINT ( 'NONE',  ( -13.27898586450066709, 3.000000000000000000, 5.170206418547661720 ) ) ;
#1471=DIRECTION ( 'NONE',  ( 0.000000000000000000, 0.000000000000000000, 1.000000000000000000 ) ) ;
#1474=ORIENTED_EDGE ( 'NONE', *, *, #6168, .F. ) ;
#1477=EDGE_CURVE ( 'NONE', #10812, #4058, #6302, .T. ) ;
#1482=CARTESIAN_POINT ( 'NONE',  ( 7.077546079049268357, 0.000000000000000000, 10.67828022838850544 ) ) ;
#1487=ORIENTED_EDGE ( 'NONE', *, *, #4130, .T. ) ;
#1488=CARTESIAN_POINT ( 'NONE',  ( 31.00000000000000000, 0.000000000000000000, 3.999999998926329514 ) ) ;
#1490=B_SPLINE_CURVE_WITH_KNOTS ( 'NONE', 3,
 ( #12693, #9306, #7309, #3097 ),
 .UNSPECIFIED., .F., .F.,
 ( 4, 4 ),
 ( 0.1547128134717859205, 1.000000000000000000 ),
 .UNSPECIFIED. ) ;
#1492=CARTESIAN_POINT ( 'NONE',  ( -13.50845331674225847, 0.000000000000000000, 1.119409668803372115 ) ) ;
#1493=DIRECTION ( 'NONE',  ( -0.000000000000000000, -1.000000000000000000, -0.000000000000000000 ) ) ;
#1500=EDGE_LOOP ( 'NONE', ( #6553, #10140, #4999, #10132 ) ) ;
#1501=VERTEX_POINT ( 'NONE', #5885 ) ;
#1508=FACE_BOUND ( 'NONE', #561, .T. ) ;
#1512=FACE_OUTER_BOUND ( 'NONE', #6478, .T. ) ;
#1518=ADVANCED_FACE ( 'NONE', ( #9124 ), #2773, .F. ) ;
#1523=ORIENTED_EDGE ( 'NONE', *, *, #12902, .T. ) ;
#1525=CARTESIAN_POINT ( 'NONE',  ( 0.000000000000000000, 3.000000000000000000, 0.000000000000000000 ) ) ;
#1526=EDGE_CURVE ( 'NONE', #12590, #8924, #3816, .T. ) ;
#1527=CARTESIAN_POINT ( 'NONE',  ( -12.14623037080100865, 3.000000000000000000, 4.072642252455982437 ) ) ;
#1528=CARTESIAN_POINT ( 'NONE',  ( 0.000000000000000000, 3.000000000000000000, 0.000000000000000000 ) ) ;
#1530=CARTESIAN_POINT ( 'NONE',  ( 2.161962830978677363, 3.000000000000000000, 14.08504230442587613 ) ) ;
#1534=DIRECTION ( 'NONE',  ( 0.000000000000000000, 0.000000000000000000, 1.000000000000000000 ) ) ;
#1539=AXIS2_PLACEMENT_3D ( 'NONE', #10224, #11328, #797 ) ;
#1541=EDGE_CURVE ( 'NONE', #10087, #357, #309, .T. ) ;
#1552=AXIS2_PLACEMENT_3D ( 'NONE', #10406, #12287, #12356 ) ;
#1556=B_SPLINE_CURVE_WITH_KNOTS ( 'NONE', 3,
 ( #3713, #1527, #1595, #1464 ),
 .UNSPECIFIED., .F., .F.,
 ( 4, 4 ),
 ( 0.1547128134717859205, 1.000000000000000000 ),
 .UNSPECIFIED. ) ;
#1557=ORIENTED_EDGE ( 'NONE', *, *, #5493, .F. ) ;
#1560=AXIS2_PLACEMENT_3D ( 'NONE', #9654, #5449, #13085 ) ;
#1562=CARTESIAN_POINT ( 'NONE',  ( -10.34346111134701118, 3.000000000000000000, -8.760376775873707444 ) ) ;
#1563=CARTESIAN_POINT ( 'NONE',  ( 11.11702303352196708, 3.000000000000000000, 8.914835885878218846 ) ) ;
#1572=ORIENTED_EDGE ( 'NONE', *, *, #10096, .T. ) ;
#1574=ORIENTED_EDGE ( 'NONE', *, *, #1526, .F. ) ;
#1583=ADVANCED_FACE ( 'NONE', ( #10520 ), #12251, .F. ) ;
#1587=VECTOR ( 'NONE', #7081, 1000.000000000000000 ) ;
#1588=ORIENTED_EDGE ( 'NONE', *, *, #788, .F. ) ;
#1591=ORIENTED_EDGE ( 'NONE', *, *, #7324, .F. ) ;
#1595=CARTESIAN_POINT ( 'NONE',  ( -12.75843939030334795, 3.000000000000000000, 4.577511697546079006 ) ) ;
#1596=CARTESIAN_POINT ( 'NONE',  ( 1.119409668803368119, 0.000000000000000000, 13.50845331674225847 ) ) ;
#1598=DIRECTION ( 'NONE',  ( 0.000000000000000000, 0.000000000000000000, 1.000000000000000000 ) ) ;
#1603=ADVANCED_FACE ( 'NONE', ( #4822 ), #13559, .T. ) ;
#1607=B_SPLINE_SURFACE_WITH_KNOTS ( 'NONE', 3, 1, ( 
 ( #7924, #2832 ),
 ( #9920, #3719 ),
 ( #8889, #11106 ),
 ( #4973, #6974 ) ),
 .UNSPECIFIED., .F., .F., .F.,
 ( 4, 4 ),
 ( 2, 2 ),
 ( 0.1547128134717859205, 1.000000000000000000 ),
 ( 0.000000000000000000, 1.000000000000000000 ),
 .UNSPECIFIED. ) ;
#1616=DIRECTION ( 'NONE',  ( -0.000000000000000000, -1.000000000000000000, -0.000000000000000000 ) ) ;
#1617=FACE_OUTER_BOUND ( 'NONE', #13568, .T. ) ;
#1618=DIRECTION ( 'NONE',  ( 0.000000000000000000, 1.000000000000000000, 0.000000000000000000 ) ) ;
#1620=EDGE_CURVE ( 'NONE', #1235, #3720, #13225, .T. ) ;
#1632=ORIENTED_EDGE ( 'NONE', *, *, #5222, .T. ) ;
#1633=CARTESIAN_POINT ( 'NONE',  ( 8.922136023539611216, 3.000000000000000000, -8.158651161643899030 ) ) ;
#1634=VECTOR ( 'NONE', #7068, 1000.000000000000000 ) ;
#1644=CARTESIAN_POINT ( 'NONE',  ( 12.03251085770905959, 3.000000000000000000, 3.999999998926332179 ) ) ;
#1645=AXIS2_PLACEMENT_3D ( 'NONE', #9835, #7977, #5911 ) ;
#1652=CARTESIAN_POINT ( 'NONE',  ( -2.604531154829235362, 3.000000000000000000, -11.80612203322752585 ) ) ;
#1655=EDGE_CURVE ( 'NONE', #8384, #1142, #4469, .T. ) ;
#1656=CARTESIAN_POINT ( 'NONE',  ( 13.04554897075798081, 3.000000000000000000, -5.733772933379503556 ) ) ;
#1663=ORIENTED_EDGE ( 'NONE', *, *, #1875, .F. ) ;
#1666=ORIENTED_EDGE ( 'NONE', *, *, #10488, .F. ) ;
#1682=B_SPLINE_SURFACE_WITH_KNOTS ( 'NONE', 3, 1, ( 
 ( #1982, #5011 ),
 ( #948, #7285 ),
 ( #9206, #3968 ),
 ( #880, #11482 ) ),
 .UNSPECIFIED., .F., .F., .F.,
 ( 4, 4 ),
 ( 2, 2 ),
 ( 0.1547128134717859205, 1.000000000000000000 ),
 ( 0.000000000000000000, 1.000000000000000000 ),
 .UNSPECIFIED. ) ;
#1687=CARTESIAN_POINT ( 'NONE',  ( -8.158651161643904359, 3.000000000000000000, -8.922136023539605887 ) ) ;
#1688=DIRECTION ( 'NONE',  ( 0.000000000000000000, 0.000000000000000000, 1.000000000000000000 ) ) ;
#1692=CARTESIAN_POINT ( 'NONE',  ( -12.07793442604884682, 3.000000000000000000, 0.5400000000005513723 ) ) ;
#1699=EDGE_LOOP ( 'NONE', ( #7649, #403, #11036, #4720 ) ) ;
#1701=EDGE_CURVE ( 'NONE', #2851, #9443, #5618, .T. ) ;
#1703=B_SPLINE_CURVE_WITH_KNOTS ( 'NONE', 3,
 ( #270, #7695, #7637, #2257 ),
 .UNSPECIFIED., .F., .F.,
 ( 4, 4 ),
 ( 0.1547128134717859205, 1.000000000000000000 ),
 .UNSPECIFIED. ) ;
#1704=CARTESIAN_POINT ( 'NONE',  ( -8.430890348300632553, 3.000000000000000000, -11.48836750521723538 ) ) ;
#1707=CARTESIAN_POINT ( 'NONE',  ( -13.33579367773357482, 3.000000000000000000, 2.428572470324200427 ) ) ;
#1709=DIRECTION ( 'NONE',  ( -0.000000000000000000, -1.000000000000000000, -0.000000000000000000 ) ) ;
#1710=CARTESIAN_POINT ( 'NONE',  ( 8.158651161643900807, 0.000000000000000000, 8.922136023539609440 ) ) ;
#1713=ORIENTED_EDGE ( 'NONE', *, *, #986, .F. ) ;
#1715=CARTESIAN_POINT ( 'NONE',  ( -2.546103534247749600, 0.000000000000000000, 12.55526518755974585 ) ) ;
#1717=ORIENTED_EDGE ( 'NONE', *, *, #4452, .T. ) ;
#1725=CARTESIAN_POINT ( 'NONE',  ( 0.000000000000000000, 3.000000000000000000, 0.000000000000000000 ) ) ;
#1727=CARTESIAN_POINT ( 'NONE',  ( -5.571433138827826426, 0.000000000000000000, -10.72973591378220526 ) ) ;
#1728=VERTEX_POINT ( 'NONE', #4320 ) ;
#1730=ORIENTED_EDGE ( 'NONE', *, *, #5620, .T. ) ;
#1734=VERTEX_POINT ( 'NONE', #194 ) ;
#1735=CARTESIAN_POINT ( 'NONE',  ( -10.69794375946289655, 3.000000000000000000, -7.065816209474156118 ) ) ;
#1737=CARTESIAN_POINT ( 'NONE',  ( -8.922226997226788470, 3.000000000000000000, -8.158551673544387484 ) ) ;
#1745=ORIENTED_EDGE ( 'NONE', *, *, #9649, .F. ) ;
#1746=DIRECTION ( 'NONE',  ( -0.000000000000000000, -1.000000000000000000, -0.000000000000000000 ) ) ;
#1753=CARTESIAN_POINT ( 'NONE',  ( 0.5400000000008001733, 3.000000000000000000, 12.07793442604883616 ) ) ;
#1756=CARTESIAN_POINT ( 'NONE',  ( -8.430890348300632553, 3.000000000000000000, -11.48836750521723538 ) ) ;
#1757=CARTESIAN_POINT ( 'NONE',  ( -3.647599401157625376, 0.000000000000000000, -11.52662650599085836 ) ) ;
#1760=EDGE_LOOP ( 'NONE', ( #6272, #5206, #5825, #4814 ) ) ;
#1764=CARTESIAN_POINT ( 'NONE',  ( 11.46814821560793618, 0.000000000000000000, -5.731782959214992701 ) ) ;
#1765=DIRECTION ( 'NONE',  ( -0.000000000000000000, -1.000000000000000000, -0.000000000000000000 ) ) ;
#1767=CIRCLE ( 'NONE', #7482, 12.08999999999737440 ) ;
#1774=CARTESIAN_POINT ( 'NONE',  ( 11.46814821560793618, 3.000000000000000000, -5.731782959214992701 ) ) ;
#1775=ORIENTED_EDGE ( 'NONE', *, *, #5333, .F. ) ;
#1777=ORIENTED_EDGE ( 'NONE', *, *, #9452, .F. ) ;
#1779=VECTOR ( 'NONE', #13132, 1000.000000000000000 ) ;
#1784=DIRECTION ( 'NONE',  ( -0.000000000000000000, -1.000000000000000000, -0.000000000000000000 ) ) ;
#1786=CARTESIAN_POINT ( 'NONE',  ( -10.33484986938308303, 3.000000000000000000, 8.771102293099071190 ) ) ;
#1789=CARTESIAN_POINT ( 'NONE',  ( -4.564691384634503635, 0.000000000000000000, 12.76342233970727769 ) ) ;
#1790=AXIS2_PLACEMENT_3D ( 'NONE', #7701, #11913, #2544 ) ;
#1793=CARTESIAN_POINT ( 'NONE',  ( 0.000000000000000000, 3.000000000000000000, 0.000000000000000000 ) ) ;
#1797=ORIENTED_EDGE ( 'NONE', *, *, #11017, .T. ) ;
#1799=EDGE_CURVE ( 'NONE', #9584, #13244, #5679, .T. ) ;
#1800=VERTEX_POINT ( 'NONE', #1633 ) ;
#1805=CARTESIAN_POINT ( 'NONE',  ( 0.000000000000000000, 3.000000000000000000, 0.000000000000000000 ) ) ;
#1807=CARTESIAN_POINT ( 'NONE',  ( -14.16466328168009881, 0.000000000000000000, 1.557181465540760534 ) ) ;
#1810=VERTEX_POINT ( 'NONE', #8771 ) ;
#1812=CARTESIAN_POINT ( 'NONE',  ( -5.571313494980134173, 3.000000000000000000, 10.72979803820131295 ) ) ;
#1816=CARTESIAN_POINT ( 'NONE',  ( -5.571433138827826426, 3.000000000000000000, -10.72973591378220526 ) ) ;
#1817=ORIENTED_EDGE ( 'NONE', *, *, #11409, .F. ) ;
#1820=CARTESIAN_POINT ( 'NONE',  ( -11.80615107470192804, 3.000000000000000000, -2.604399508764160487 ) ) ;
#1826=DIRECTION ( 'NONE',  ( 0.000000000000000000, 1.000000000000000000, 0.000000000000000000 ) ) ;
#1833=CARTESIAN_POINT ( 'NONE',  ( -8.158651161643904359, 3.000000000000000000, -8.922136023539605887 ) ) ;
#1836=ORIENTED_EDGE ( 'NONE', *, *, #303, .F. ) ;
#1839=CARTESIAN_POINT ( 'NONE',  ( 8.158651161643900807, 0.000000000000000000, 8.922136023539609440 ) ) ;
#1846=CARTESIAN_POINT ( 'NONE',  ( -12.79759916868914615, 3.000000000000000000, -0.7702044561450367421 ) ) ;
#1847=CARTESIAN_POINT ( 'NONE',  ( -0.7702044561450404059, 0.000000000000000000, 12.79759916868914793 ) ) ;
#1848=ORIENTED_EDGE ( 'NONE', *, *, #5747, .F. ) ;
#1852=VECTOR ( 'NONE', #9576, 1000.000000000000000 ) ;
#1855=CARTESIAN_POINT ( 'NONE',  ( -2.161962830978785277, 0.000000000000000000, -14.08504230442586369 ) ) ;
#1858=CARTESIAN_POINT ( 'NONE',  ( 7.712570079660896916, 3.000000000000000000, -11.14709020439929432 ) ) ;
#1861=AXIS2_PLACEMENT_3D ( 'NONE', #5283, #260, #9485 ) ;
#1864=VERTEX_POINT ( 'NONE', #9049 ) ;
#1871=CARTESIAN_POINT ( 'NONE',  ( 8.430890348300586368, 0.000000000000000000, -11.48836750521726913 ) ) ;
#1874=VECTOR ( 'NONE', #12257, 1000.000000000000000 ) ;
#1875=EDGE_CURVE ( 'NONE', #9276, #10087, #11385, .T. ) ;
#1887=VERTEX_POINT ( 'NONE', #7952 ) ;
#1891=ADVANCED_FACE ( 'NONE', ( #12099 ), #351, .F. ) ;
#1896=CARTESIAN_POINT ( 'NONE',  ( 13.04554897075798081, 0.000000000000000000, -5.733772933379503556 ) ) ;
#1898=CARTESIAN_POINT ( 'NONE',  ( -5.784789447945489549, 0.000000000000000000, 12.25836857253663581 ) ) ;
#1900=B_SPLINE_SURFACE_WITH_KNOTS ( 'NONE', 3, 1, ( 
 ( #5211, #9268 ),
 ( #874, #9548 ),
 ( #6073, #8362 ),
 ( #8162, #12392 ) ),
 .UNSPECIFIED., .F., .F., .F.,
 ( 4, 4 ),
 ( 2, 2 ),
 ( 0.000000000000000000, 0.8452273900860258760 ),
 ( 0.000000000000000000, 1.000000000000000000 ),
 .UNSPECIFIED. ) ;
#1902=FACE_OUTER_BOUND ( 'NONE', #353, .T. ) ;
#1903=DIRECTION ( 'NONE',  ( -0.000000000000000000, -1.000000000000000000, -0.000000000000000000 ) ) ;
#1904=DIRECTION ( 'NONE',  ( -0.000000000000000000, -1.000000000000000000, -0.000000000000000000 ) ) ;
#1905=CARTESIAN_POINT ( 'NONE',  ( 10.72973591378220704, 3.000000000000000000, -5.571433138827823761 ) ) ;
#1909=EDGE_LOOP ( 'NONE', ( #12844, #5302, #9727, #3674 ) ) ;
#1911=ADVANCED_FACE ( 'NONE', ( #7749 ), #10138, .F. ) ;
#1912=ORIENTED_EDGE ( 'NONE', *, *, #6042, .F. ) ;
#1917=DIRECTION ( 'NONE',  ( 0.000000000000000000, 1.000000000000000000, 0.000000000000000000 ) ) ;
#1920=CARTESIAN_POINT ( 'NONE',  ( 0.000000000000000000, 0.000000000000000000, 0.000000000000000000 ) ) ;
#1924=VERTEX_POINT ( 'NONE', #1488 ) ;
#1925=CARTESIAN_POINT ( 'NONE',  ( 8.922136023539611216, 0.000000000000000000, -8.158651161643899030 ) ) ;
#1927=CARTESIAN_POINT ( 'NONE',  ( -12.16218796965919324, 0.000000000000000000, -4.056222772158363021 ) ) ;
#1930=DIRECTION ( 'NONE',  ( 0.000000000000000000, 1.000000000000000000, 0.000000000000000000 ) ) ;
#1931=ORIENTED_EDGE ( 'NONE', *, *, #3127, .T. ) ;
#1933=VERTEX_POINT ( 'NONE', #8838 ) ;
#1935=CARTESIAN_POINT ( 'NONE',  ( 0.000000000000000000, 3.000000000000000000, 0.000000000000000000 ) ) ;
#1943=CARTESIAN_POINT ( 'NONE',  ( 11.11702303352194043, 0.000000000000000000, -8.914835885878249044 ) ) ;
#1944=ORIENTED_EDGE ( 'NONE', *, *, #2600, .F. ) ;
#1947=ORIENTED_EDGE ( 'NONE', *, *, #12833, .T. ) ;
#1955=CARTESIAN_POINT ( 'NONE',  ( -12.56087513340552242, 3.000000000000000000, 2.568302020731519253 ) ) ;
#1963=CARTESIAN_POINT ( 'NONE',  ( 0.000000000000000000, 3.000000000000000000, 0.000000000000000000 ) ) ;
#1967=ORIENTED_EDGE ( 'NONE', *, *, #8053, .T. ) ;
#1971=EDGE_LOOP ( 'NONE', ( #10807, #2206, #785, #12247 ) ) ;
#1976=CARTESIAN_POINT ( 'NONE',  ( -8.430890348300124515, 3.000000000000000000, 11.48836750521761019 ) ) ;
#1979=CARTESIAN_POINT ( 'NONE',  ( -1.557181465540677712, 0.000000000000000000, 14.16466328168010769 ) ) ;
#1982=CARTESIAN_POINT ( 'NONE',  ( 10.72979803820132005, 3.000000000000000000, 5.571313494980133285 ) ) ;
#1983=ORIENTED_EDGE ( 'NONE', *, *, #5070, .F. ) ;
#1986=DIRECTION ( 'NONE',  ( 0.000000000000000000, 1.000000000000000000, 0.000000000000000000 ) ) ;
#1988=CARTESIAN_POINT ( 'NONE',  ( 0.7702044561450380744, 3.000000000000000000, -12.79759916868914615 ) ) ;
#1991=EDGE_CURVE ( 'NONE', #781, #2012, #11343, .T. ) ;
#1995=VECTOR ( 'NONE', #12447, 1000.000000000000000 ) ;
#1997=AXIS2_PLACEMENT_3D ( 'NONE', #12007, #8886, #3511 ) ;
#1999=CYLINDRICAL_SURFACE ( 'NONE', #9067, 14.25000000000000000 ) ;
#2003=CARTESIAN_POINT ( 'NONE',  ( -6.506507307819711095, 0.000000000000000000, 10.18987059060247624 ) ) ;
#2006=B_SPLINE_CURVE_WITH_KNOTS ( 'NONE', 3,
 ( #9525, #172, #106, #4288 ),
 .UNSPECIFIED., .F., .F.,
 ( 4, 4 ),
 ( 0.1547128134717859205, 0.7774895956119340923 ),
 .UNSPECIFIED. ) ;
#2012=VERTEX_POINT ( 'NONE', #3003 ) ;
#2021=DIRECTION ( 'NONE',  ( 0.000000000000000000, 1.000000000000000000, 0.000000000000000000 ) ) ;
#2027=CARTESIAN_POINT ( 'NONE',  ( -14.08504230442586369, 3.000000000000000000, 2.161962830978781724 ) ) ;
#2032=ORIENTED_EDGE ( 'NONE', *, *, #11788, .F. ) ;
#2036=EDGE_LOOP ( 'NONE', ( #416, #5647, #158, #8553 ) ) ;
#2037=LINE ( 'NONE', #1009, #527 ) ;
#2038=DIRECTION ( 'NONE',  ( 0.000000000000000000, 0.000000000000000000, -1.000000000000000000 ) ) ;
#2040=FACE_OUTER_BOUND ( 'NONE', #3559, .T. ) ;
#2041=APPLICATION_CONTEXT ( 'automotive_design' ) ;
#2042=CARTESIAN_POINT ( 'NONE',  ( 0.7702044561450380744, 3.000000000000000000, -12.79759916868914615 ) ) ;
#2053=AXIS2_PLACEMENT_3D ( 'NONE', #13357, #4804, #5841 ) ;
#2057=LINE ( 'NONE', #8572, #5961 ) ;
#2059=CARTESIAN_POINT ( 'NONE',  ( -9.593885948927676210, 3.000000000000000000, 8.504652361247165615 ) ) ;
#2062=VECTOR ( 'NONE', #7421, 1000.000000000000000 ) ;
#2066=VERTEX_POINT ( 'NONE', #5134 ) ;
#2071=EDGE_CURVE ( 'NONE', #10341, #8124, #2037, .T. ) ;
#2072=EDGE_CURVE ( 'NONE', #5132, #3799, #6297, .T. ) ;
#2074=AXIS2_PLACEMENT_3D ( 'NONE', #10610, #10742, #9502 ) ;
#2075=CARTESIAN_POINT ( 'NONE',  ( 5.733772933379474246, 0.000000000000000000, -13.04554897075799502 ) ) ;
#2076=VECTOR ( 'NONE', #10909, 1000.000000000000000 ) ;
#2077=CARTESIAN_POINT ( 'NONE',  ( 0.000000000000000000, 3.000000000000000000, 0.000000000000000000 ) ) ;
#2083=VERTEX_POINT ( 'NONE', #1839 ) ;
#2084=CIRCLE ( 'NONE', #1645, 14.25000000000000178 ) ;
#2087=CARTESIAN_POINT ( 'NONE',  ( 0.000000000000000000, 0.000000000000000000, 0.000000000000000000 ) ) ;
#2089=CARTESIAN_POINT ( 'NONE',  ( -5.733772933379540859, 0.000000000000000000, -13.04554897075796660 ) ) ;
#2090=DIRECTION ( 'NONE',  ( 0.000000000000000000, 0.000000000000000000, -1.000000000000000000 ) ) ;
#2098=FACE_OUTER_BOUND ( 'NONE', #1133, .T. ) ;
#2104=VERTEX_POINT ( 'NONE', #3325 ) ;
#2111=CARTESIAN_POINT ( 'NONE',  ( -3.647470871583628593, 0.000000000000000000, 11.52666717836884125 ) ) ;
#2116=DIRECTION ( 'NONE',  ( 0.000000000000000000, 0.000000000000000000, -1.000000000000000000 ) ) ;
#2120=DIRECTION ( 'NONE',  ( -0.000000000000000000, -1.000000000000000000, -0.000000000000000000 ) ) ;
#2126=LINE ( 'NONE', #11835, #8430 ) ;
#2131=CARTESIAN_POINT ( 'NONE',  ( -0.5398653231797316820, 3.000000000000000000, 12.07794044664754018 ) ) ;
#2138=DIRECTION ( 'NONE',  ( -0.000000000000000000, -1.000000000000000000, -0.000000000000000000 ) ) ;
#2148=B_SPLINE_CURVE_WITH_KNOTS ( 'NONE', 3,
 ( #6724, #333, #6658, #3621 ),
 .UNSPECIFIED., .F., .F.,
 ( 4, 4 ),
 ( 0.1547128134717859205, 1.000000000000000000 ),
 .UNSPECIFIED. ) ;
#2152=CARTESIAN_POINT ( 'NONE',  ( 8.914835885878220623, 3.000000000000000000, -11.11702303352196708 ) ) ;
#2155=CARTESIAN_POINT ( 'NONE',  ( -2.546103534247749600, 0.000000000000000000, 12.55526518755974585 ) ) ;
#2157=B_SPLINE_SURFACE_WITH_KNOTS ( 'NONE', 3, 1, ( 
 ( #3066, #7343 ),
 ( #5141, #6438 ),
 ( #4309, #7474 ),
 ( #12654, #6300 ) ),
 .UNSPECIFIED., .F., .F., .F.,
 ( 4, 4 ),
 ( 2, 2 ),
 ( 0.1547128134717859205, 1.000000000000000000 ),
 ( 0.000000000000000000, 1.000000000000000000 ),
 .UNSPECIFIED. ) ;
#2160=ORIENTED_EDGE ( 'NONE', *, *, #61, .T. ) ;
#2166=ORIENTED_EDGE ( 'NONE', *, *, #8840, .F. ) ;
#2180=DIRECTION ( 'NONE',  ( -0.000000000000000000, -1.000000000000000000, -0.000000000000000000 ) ) ;
#2182=CARTESIAN_POINT ( 'NONE',  ( 2.604531154829233586, 0.000000000000000000, 11.80612203322752585 ) ) ;
#2183=AXIS2_PLACEMENT_3D ( 'NONE', #6797, #9897, #6873 ) ;
#2188=ORIENTED_EDGE ( 'NONE', *, *, #4381, .F. ) ;
#2194=EDGE_CURVE ( 'NONE', #9874, #11321, #682, .T. ) ;
#2198=CARTESIAN_POINT ( 'NONE',  ( 0.000000000000000000, 3.000000000000000000, 0.000000000000000000 ) ) ;
#2201=AXIS2_PLACEMENT_3D ( 'NONE', #1240, #5431, #12 ) ;
#2205=( NAMED_UNIT ( * ) SI_UNIT ( $, .STERADIAN. ) SOLID_ANGLE_UNIT ( ) );
#2206=ORIENTED_EDGE ( 'NONE', *, *, #6575, .F. ) ;
#2208=VERTEX_POINT ( 'NONE', #7409 ) ;
#2211=B_SPLINE_CURVE_WITH_KNOTS ( 'NONE', 3,
 ( #169, #5586, #11930, #4557 ),
 .UNSPECIFIED., .F., .F.,
 ( 4, 4 ),
 ( 0.1547128134717859205, 1.000000000000000000 ),
 .UNSPECIFIED. ) ;
#2215=FACE_OUTER_BOUND ( 'NONE', #10799, .T. ) ;
#2221=DIRECTION ( 'NONE',  ( -0.000000000000000000, -1.000000000000000000, -0.000000000000000000 ) ) ;
#2227=ORIENTED_EDGE ( 'NONE', *, *, #3550, .F. ) ;
#2228=EDGE_LOOP ( 'NONE', ( #10791, #2911, #11622, #2887 ) ) ;
#2230=DIRECTION ( 'NONE',  ( 0.000000000000000000, 0.000000000000000000, -1.000000000000000000 ) ) ;
#2238=ORIENTED_EDGE ( 'NONE', *, *, #4761, .F. ) ;
#2241=B_SPLINE_SURFACE_WITH_KNOTS ( 'NONE', 3, 1, ( 
 ( #13553, #1979 ),
 ( #10311, #7009 ),
 ( #4941, #1847 ),
 ( #10168, #13279 ) ),
 .UNSPECIFIED., .F., .F., .F.,
 ( 4, 4 ),
 ( 2, 2 ),
 ( 0.000000000000000000, 0.8452273900860258760 ),
 ( 0.000000000000000000, 1.000000000000000000 ),
 .UNSPECIFIED. ) ;
#2242=ORIENTED_EDGE ( 'NONE', *, *, #11661, .T. ) ;
#2249=DIRECTION ( 'NONE',  ( 0.000000000000000000, 1.000000000000000000, 0.000000000000000000 ) ) ;
#2256=ORIENTED_EDGE ( 'NONE', *, *, #4060, .F. ) ;
#2257=CARTESIAN_POINT ( 'NONE',  ( 1.557181465540758758, 0.000000000000000000, 14.16466328168009881 ) ) ;
#2259=AXIS2_PLACEMENT_3D ( 'NONE', #4077, #5105, #11443 ) ;
#2264=VECTOR ( 'NONE', #6097, 1000.000000000000000 ) ;
#2265=LINE ( 'NONE', #349, #1852 ) ;
#2271=DIRECTION ( 'NONE',  ( -0.000000000000000000, -1.000000000000000000, -0.000000000000000000 ) ) ;
#2289=CARTESIAN_POINT ( 'NONE',  ( -8.158551673544545579, 0.000000000000000000, 8.922226997226644585 ) ) ;
#2291=LINE ( 'NONE', #6494, #9092 ) ;
#2295=AXIS2_PLACEMENT_3D ( 'NONE', #11971, #1709, #668 ) ;
#2308=AXIS2_PLACEMENT_3D ( 'NONE', #10702, #2567, #6698 ) ;
#2315=CARTESIAN_POINT ( 'NONE',  ( 0.000000000000000000, 3.000000000000000000, 0.000000000000000000 ) ) ;
#2319=EDGE_LOOP ( 'NONE', ( #8530, #11983, #7800, #3488 ) ) ;
#2323=SHAPE_REPRESENTATION ( 'gear-link-1', ( #10007 ), #5843 ) ;
#2332=CARTESIAN_POINT ( 'NONE',  ( 4.072642252455978884, 3.000000000000000000, 12.14623037080101042 ) ) ;
#2334=EDGE_CURVE ( 'NONE', #9307, #12420, #4570, .T. ) ;
#2338=CARTESIAN_POINT ( 'NONE',  ( 8.914835885878215294, 3.000000000000000000, 11.11702303352197418 ) ) ;
#2340=DIRECTION ( 'NONE',  ( 0.000000000000000000, 1.000000000000000000, 0.000000000000000000 ) ) ;
#2342=CARTESIAN_POINT ( 'NONE',  ( -11.48836750521723893, 3.000000000000000000, 8.430890348300625448 ) ) ;
#2345=CYLINDRICAL_SURFACE ( 'NONE', #562, 12.08999999999737440 ) ;
#2346=EDGE_CURVE ( 'NONE', #3691, #8949, #4938, .T. ) ;
#2347=VERTEX_POINT ( 'NONE', #7802 ) ;
#2350=ORIENTED_EDGE ( 'NONE', *, *, #6212, .T. ) ;
#2360=CARTESIAN_POINT ( 'NONE',  ( 2.414978278956333213, 0.000000000000000000, -13.33788847341978645 ) ) ;
#2362=DIRECTION ( 'NONE',  ( 0.000000000000000000, 0.000000000000000000, 1.000000000000000000 ) ) ;
#2364=EDGE_LOOP ( 'NONE', ( #8853, #13343, #7550, #4962 ) ) ;
#2367=B_SPLINE_SURFACE_WITH_KNOTS ( 'NONE', 3, 1, ( 
 ( #13220, #4683 ),
 ( #4609, #12203 ),
 ( #12060, #11157 ),
 ( #2754, #1727 ) ),
 .UNSPECIFIED., .F., .F., .F.,
 ( 4, 4 ),
 ( 2, 2 ),
 ( 0.000000000000000000, 0.8452273900860258760 ),
 ( 0.000000000000000000, 1.000000000000000000 ),
 .UNSPECIFIED. ) ;
#2369=CIRCLE ( 'NONE', #5444, 12.08999999999737440 ) ;
#2375=CARTESIAN_POINT ( 'NONE',  ( -0.5400000000007666445, 3.000000000000000000, -12.07793442604883793 ) ) ;
#2377=CARTESIAN_POINT ( 'NONE',  ( 0.000000000000000000, 3.000000000000000000, 0.000000000000000000 ) ) ;
#2383=B_SPLINE_CURVE_WITH_KNOTS ( 'NONE', 3,
 ( #2089, #12566, #11452, #6218 ),
 .UNSPECIFIED., .F., .F.,
 ( 4, 4 ),
 ( 0.000000000000000000, 0.8452273900860258760 ),
 .UNSPECIFIED. ) ;
#2387=DIRECTION ( 'NONE',  ( 0.000000000000000000, 0.000000000000000000, -1.000000000000000000 ) ) ;
#2389=DIRECTION ( 'NONE',  ( -0.000000000000000000, -1.000000000000000000, -0.000000000000000000 ) ) ;
#2390=DIRECTION ( 'NONE',  ( 0.000000000000000000, 1.000000000000000000, 0.000000000000000000 ) ) ;
#2406=DIRECTION ( 'NONE',  ( -0.000000000000000000, -1.000000000000000000, -0.000000000000000000 ) ) ;
#2421=CARTESIAN_POINT ( 'NONE',  ( 8.430890348300586368, 3.000000000000000000, -11.48836750521726913 ) ) ;
#2422=CARTESIAN_POINT ( 'NONE',  ( -13.04554897075795949, 0.000000000000000000, 5.733772933379550629 ) ) ;
#2429=AXIS2_PLACEMENT_3D ( 'NONE', #1528, #5587, #2618 ) ;
#2433=CARTESIAN_POINT ( 'NONE',  ( -5.708888906988910605, 0.000000000000000000, 11.46847481510586597 ) ) ;
#2440=VECTOR ( 'NONE', #9770, 1000.000000000000000 ) ;
#2441=LINE ( 'NONE', #7810, #10166 ) ;
#2447=EDGE_CURVE ( 'NONE', #9461, #8060, #5112, .T. ) ;
#2449=CARTESIAN_POINT ( 'NONE',  ( -11.11702303352192445, 0.000000000000000000, 8.914835885878272137 ) ) ;
#2452=CARTESIAN_POINT ( 'NONE',  ( -11.11702303352197063, 3.000000000000000000, -8.914835885878215294 ) ) ;
#2453=ADVANCED_FACE ( 'NONE', ( #11389 ), #9801, .F. ) ;
#2455=CARTESIAN_POINT ( 'NONE',  ( -1.119409668803374558, 3.000000000000000000, -13.50845331674225669 ) ) ;
#2456=CARTESIAN_POINT ( 'NONE',  ( 12.01285915242476499, 0.000000000000000000, -4.000000001073668265 ) ) ;
#2457=VECTOR ( 'NONE', #2831, 1000.000000000000000 ) ;
#2459=CARTESIAN_POINT ( 'NONE',  ( 13.27898586450067242, 0.000000000000000000, -5.170206418547655502 ) ) ;
#2460=ORIENTED_EDGE ( 'NONE', *, *, #12770, .F. ) ;
#2466=ORIENTED_EDGE ( 'NONE', *, *, #7621, .F. ) ;
#2468=CIRCLE ( 'NONE', #13473, 12.08999999999737440 ) ;
#2469=CARTESIAN_POINT ( 'NONE',  ( -5.733772933379472470, 3.000000000000000000, 13.04554897075799502 ) ) ;
#2478=CARTESIAN_POINT ( 'NONE',  ( 31.00000000000000000, 3.000000000000000000, -1.073670993220974656E-09 ) ) ;
#2484=EDGE_CURVE ( 'NONE', #8093, #9473, #8242, .T. ) ;
#2486=ORIENTED_EDGE ( 'NONE', *, *, #1201, .T. ) ;
#2502=VERTEX_POINT ( 'NONE', #11794 ) ;
#2503=VECTOR ( 'NONE', #6003, 1000.000000000000000 ) ;
#2504=CIRCLE ( 'NONE', #4036, 14.25000000000000178 ) ;
#2510=CARTESIAN_POINT ( 'NONE',  ( 10.18987059060247269, 3.000000000000000000, 6.506507307819714647 ) ) ;
#2514=CARTESIAN_POINT ( 'NONE',  ( -2.414978278956346092, 3.000000000000000000, 13.33788847341978467 ) ) ;
#2522=CARTESIAN_POINT ( 'NONE',  ( -8.914835885878215294, 3.000000000000000000, 11.11702303352197063 ) ) ;
#2526=CARTESIAN_POINT ( 'NONE',  ( -12.25282671965375236, 3.000000000000000000, 5.797378255456025364 ) ) ;
#2534=ORIENTED_EDGE ( 'NONE', *, *, #6327, .F. ) ;
#2537=CARTESIAN_POINT ( 'NONE',  ( -13.27898586450070084, 3.000000000000000000, -5.170206418547588001 ) ) ;
#2539=ORIENTED_EDGE ( 'NONE', *, *, #13367, .F. ) ;
#2540=COLOUR_RGB ( '',0.7803921568627451011, 0.7607843137254901578, 0.7411764705882353255 ) ;
#2544=DIRECTION ( 'NONE',  ( 0.000000000000000000, 0.000000000000000000, 1.000000000000000000 ) ) ;
#2545=CARTESIAN_POINT ( 'NONE',  ( -13.27898586450070084, 3.000000000000000000, -5.170206418547585336 ) ) ;
#2549=CARTESIAN_POINT ( 'NONE',  ( 2.428572470324196431, 0.000000000000000000, 13.33579367773357127 ) ) ;
#2552=CARTESIAN_POINT ( 'NONE',  ( 5.170206418547656391, 0.000000000000000000, 13.27898586450067064 ) ) ;
#2554=EDGE_CURVE ( 'NONE', #9891, #9128, #4353, .T. ) ;
#2555=ORIENTED_EDGE ( 'NONE', *, *, #8829, .F. ) ;
#2565=CYLINDRICAL_SURFACE ( 'NONE', #2668, 12.08999999999737440 ) ;
#2566=ADVANCED_FACE ( 'NONE', ( #2215 ), #5311, .T. ) ;
#2567=DIRECTION ( 'NONE',  ( -0.000000000000000000, -1.000000000000000000, -0.000000000000000000 ) ) ;
#2570=ORIENTED_EDGE ( 'NONE', *, *, #8684, .T. ) ;
#2584=ORIENTED_EDGE ( 'NONE', *, *, #8168, .F. ) ;
#2589=CARTESIAN_POINT ( 'NONE',  ( -11.52662650599083882, 3.000000000000000000, 3.647599401157695986 ) ) ;
#2590=CARTESIAN_POINT ( 'NONE',  ( -8.158551673544545579, 3.000000000000000000, 8.922226997226644585 ) ) ;
#2597=ORIENTED_EDGE ( 'NONE', *, *, #10550, .F. ) ;
#2599=EDGE_LOOP ( 'NONE', ( #6343, #179, #10416, #11865 ) ) ;
#2600=EDGE_CURVE ( 'NONE', #4662, #1924, #12828, .T. ) ;
#2601=CARTESIAN_POINT ( 'NONE',  ( 11.48836750521724070, 3.000000000000000000, 8.430890348300627224 ) ) ;
#2606=CYLINDRICAL_SURFACE ( 'NONE', #3781, 14.25000000000000355 ) ;
#2607=CARTESIAN_POINT ( 'NONE',  ( 2.604531154829233586, 0.000000000000000000, 11.80612203322752585 ) ) ;
#2609=ORIENTED_EDGE ( 'NONE', *, *, #11038, .F. ) ;
#2611=DIRECTION ( 'NONE',  ( -0.000000000000000000, -1.000000000000000000, -0.000000000000000000 ) ) ;
#2613=EDGE_CURVE ( 'NONE', #4963, #8964, #21, .T. ) ;
#2615=EDGE_CURVE ( 'NONE', #11718, #9350, #5511, .T. ) ;
#2618=DIRECTION ( 'NONE',  ( 0.000000000000000000, 0.000000000000000000, 1.000000000000000000 ) ) ;
#2620=CARTESIAN_POINT ( 'NONE',  ( -12.07793442604883971, 3.000000000000000000, 0.5400000000008015055 ) ) ;
#2632=DIRECTION ( 'NONE',  ( 0.000000000000000000, 1.000000000000000000, 0.000000000000000000 ) ) ;
#2639=B_SPLINE_CURVE_WITH_KNOTS ( 'NONE', 3,
 ( #8648, #11628, #1156, #4453 ),
 .UNSPECIFIED., .F., .F.,
 ( 4, 4 ),
 ( 0.1547128134717859205, 1.000000000000000000 ),
 .UNSPECIFIED. ) ;
#2641=FACE_OUTER_BOUND ( 'NONE', #9845, .T. ) ;
#2643=AXIS2_PLACEMENT_3D ( 'NONE', #3715, #7791, #7918 ) ;
#2644=ORIENTED_EDGE ( 'NONE', *, *, #2953, .F. ) ;
#2645=VERTEX_POINT ( 'NONE', #9989 ) ;
#2647=ORIENTED_EDGE ( 'NONE', *, *, #13125, .T. ) ;
#2648=CARTESIAN_POINT ( 'NONE',  ( 5.571433138827823761, 0.000000000000000000, 10.72973591378220704 ) ) ;
#2652=VECTOR ( 'NONE', #7773, 1000.000000000000000 ) ;
#2653=DIRECTION ( 'NONE',  ( 0.000000000000000000, 1.000000000000000000, 0.000000000000000000 ) ) ;
#2654=DIRECTION ( 'NONE',  ( -0.000000000000000000, -1.000000000000000000, -0.000000000000000000 ) ) ;
#2657=CYLINDRICAL_SURFACE ( 'NONE', #3605, 14.24999999999999822 ) ;
#2662=VECTOR ( 'NONE', #2711, 1000.000000000000000 ) ;
#2665=VERTEX_POINT ( 'NONE', #6816 ) ;
#2668=AXIS2_PLACEMENT_3D ( 'NONE', #2766, #13314, #8888 ) ;
#2669=EDGE_CURVE ( 'NONE', #7043, #2208, #93, .T. ) ;
#2680=ORIENTED_EDGE ( 'NONE', *, *, #6184, .T. ) ;
#2681=CARTESIAN_POINT ( 'NONE',  ( -5.170206418547658167, 3.000000000000000000, -13.27898586450066887 ) ) ;
#2683=CARTESIAN_POINT ( 'NONE',  ( 0.000000000000000000, 0.000000000000000000, 0.000000000000000000 ) ) ;
#2688=AXIS2_PLACEMENT_3D ( 'NONE', #1186, #4141, #4204 ) ;
#2701=VECTOR ( 'NONE', #12682, 1000.000000000000000 ) ;
#2711=DIRECTION ( 'NONE',  ( -0.000000000000000000, -1.000000000000000000, -0.000000000000000000 ) ) ;
#2713=VECTOR ( 'NONE', #1904, 1000.000000000000000 ) ;
#2716=CIRCLE ( 'NONE', #12192, 14.25000000000000178 ) ;
#2719=ORIENTED_EDGE ( 'NONE', *, *, #3807, .T. ) ;
#2721=ORIENTED_EDGE ( 'NONE', *, *, #4452, .F. ) ;
#2723=ORIENTED_EDGE ( 'NONE', *, *, #13134, .F. ) ;
#2724=CARTESIAN_POINT ( 'NONE',  ( 5.731782959214990036, 3.000000000000000000, 11.46814821560793618 ) ) ;
#2726=CARTESIAN_POINT ( 'NONE',  ( 7.723663868796767140, 0.000000000000000000, 11.13895890373327191 ) ) ;
#2729=CARTESIAN_POINT ( 'NONE',  ( -8.430890348300124515, 3.000000000000000000, 11.48836750521761019 ) ) ;
#2730=FACE_OUTER_BOUND ( 'NONE', #10027, .T. ) ;
#2731=EDGE_CURVE ( 'NONE', #10022, #7906, #2369, .T. ) ;
#2739=ORIENTED_EDGE ( 'NONE', *, *, #12101, .F. ) ;
#2743=CARTESIAN_POINT ( 'NONE',  ( -2.428572470324203980, 3.000000000000000000, -13.33579367773357482 ) ) ;
#2747=CARTESIAN_POINT ( 'NONE',  ( 1.557181465540669496, 0.000000000000000000, -14.16466328168010769 ) ) ;
#2748=DIRECTION ( 'NONE',  ( 0.000000000000000000, 1.000000000000000000, 0.000000000000000000 ) ) ;
#2749=LINE ( 'NONE', #13292, #4500 ) ;
#2754=CARTESIAN_POINT ( 'NONE',  ( -5.571433138827826426, 3.000000000000000000, -10.72973591378220526 ) ) ;
#2756=VECTOR ( 'NONE', #1118, 1000.000000000000000 ) ;
#2762=CARTESIAN_POINT ( 'NONE',  ( 0.000000000000000000, 3.000000000000000000, 0.000000000000000000 ) ) ;
#2766=CARTESIAN_POINT ( 'NONE',  ( 0.000000000000000000, 3.000000000000000000, 0.000000000000000000 ) ) ;
#2773=B_SPLINE_SURFACE_WITH_KNOTS ( 'NONE', 3, 1, ( 
 ( #8089, #6847 ),
 ( #11049, #8019 ),
 ( #10016, #4848 ),
 ( #12240, #13338 ) ),
 .UNSPECIFIED., .F., .F., .F.,
 ( 4, 4 ),
 ( 2, 2 ),
 ( 0.1547128134717859205, 1.000000000000000000 ),
 ( 0.000000000000000000, 1.000000000000000000 ),
 .UNSPECIFIED. ) ;
#2775=DIRECTION ( 'NONE',  ( -0.000000000000000000, -1.000000000000000000, -0.000000000000000000 ) ) ;
#2777=LINE ( 'NONE', #11117, #4290 ) ;
#2782=DIRECTION ( 'NONE',  ( 0.000000000000000000, 0.000000000000000000, 1.000000000000000000 ) ) ;
#2785=CARTESIAN_POINT ( 'NONE',  ( -0.7901945867173586491, 0.000000000000000000, -12.78643498603818074 ) ) ;
#2788=ORIENTED_EDGE ( 'NONE', *, *, #9212, .T. ) ;
#2791=CARTESIAN_POINT ( 'NONE',  ( -8.482622935103766082, 0.000000000000000000, 9.600126836553263487 ) ) ;
#2796=CARTESIAN_POINT ( 'NONE',  ( 5.733772933379453818, 3.000000000000000000, 13.04554897075800568 ) ) ;
#2799=EDGE_CURVE ( 'NONE', #12697, #9707, #6912, .T. ) ;
#2802=ORIENTED_EDGE ( 'NONE', *, *, #2554, .T. ) ;
#2806=ORIENTED_EDGE ( 'NONE', *, *, #11223, .F. ) ;
#2809=CARTESIAN_POINT ( 'NONE',  ( 0.7901945867173618687, 3.000000000000000000, 12.78643498603817541 ) ) ;
#2812=CARTESIAN_POINT ( 'NONE',  ( -8.771102293099080072, 3.000000000000000000, -10.33484986938307770 ) ) ;
#2816=APPLICATION_CONTEXT ( 'automotive_design' ) ;
#2822=CARTESIAN_POINT ( 'NONE',  ( -10.69794375946289655, 0.000000000000000000, -7.065816209474156118 ) ) ;
#2824=ORIENTED_EDGE ( 'NONE', *, *, #4997, .F. ) ;
#2831=DIRECTION ( 'NONE',  ( -0.000000000000000000, -1.000000000000000000, -0.000000000000000000 ) ) ;
#2832=CARTESIAN_POINT ( 'NONE',  ( -0.5400000000008023937, 0.000000000000000000, -12.07793442604883971 ) ) ;
#2836=EDGE_LOOP ( 'NONE', ( #12806, #8634, #12442, #5287 ) ) ;
#2840=CARTESIAN_POINT ( 'NONE',  ( 8.504652361247167391, 3.000000000000000000, 9.593885948927674434 ) ) ;
#2841=CARTESIAN_POINT ( 'NONE',  ( 10.33484986938308481, 0.000000000000000000, -8.771102293099065861 ) ) ;
#2843=CYLINDRICAL_SURFACE ( 'NONE', #4838, 4.000000000000000000 ) ;
#2844=DIRECTION ( 'NONE',  ( 0.000000000000000000, 0.000000000000000000, 1.000000000000000000 ) ) ;
#2848=CARTESIAN_POINT ( 'NONE',  ( 5.733772933379453818, 3.000000000000000000, 13.04554897075800568 ) ) ;
#2850=CARTESIAN_POINT ( 'NONE',  ( -4.072642252455976219, 3.000000000000000000, -12.14623037080101398 ) ) ;
#2851=VERTEX_POINT ( 'NONE', #2894 ) ;
#2852=VERTEX_POINT ( 'NONE', #2969 ) ;
#2853=CIRCLE ( 'NONE', #8342, 14.25000000000000355 ) ;
#2856=ORIENTED_EDGE ( 'NONE', *, *, #10469, .T. ) ;
#2869=ADVANCED_FACE ( 'NONE', ( #3030 ), #12352, .T. ) ;
#2874=EDGE_CURVE ( 'NONE', #2852, #7906, #9163, .T. ) ;
#2877=DIRECTION ( 'NONE',  ( -0.000000000000000000, -1.000000000000000000, -0.000000000000000000 ) ) ;
#2884=ORIENTED_EDGE ( 'NONE', *, *, #8769, .F. ) ;
#2887=ORIENTED_EDGE ( 'NONE', *, *, #3513, .T. ) ;
#2893=AXIS2_PLACEMENT_3D ( 'NONE', #5033, #9229, #3233 ) ;
#2894=CARTESIAN_POINT ( 'NONE',  ( -8.914835885878215294, 3.000000000000000000, 11.11702303352197063 ) ) ;
#2900=CARTESIAN_POINT ( 'NONE',  ( -13.27898586450070084, 3.000000000000000000, -5.170206418547588001 ) ) ;
#2902=ORIENTED_EDGE ( 'NONE', *, *, #5723, .T. ) ;
#2904=CARTESIAN_POINT ( 'NONE',  ( 2.161962830978694683, 0.000000000000000000, -14.08504230442587790 ) ) ;
#2909=ORIENTED_EDGE ( 'NONE', *, *, #5373, .T. ) ;
#2910=CARTESIAN_POINT ( 'NONE',  ( -11.80615107470192804, 3.000000000000000000, -2.604399508764160487 ) ) ;
#2911=ORIENTED_EDGE ( 'NONE', *, *, #13125, .F. ) ;
#2916=CIRCLE ( 'NONE', #10619, 12.08999999999737440 ) ;
#2926=ORIENTED_EDGE ( 'NONE', *, *, #11909, .F. ) ;
#2930=B_SPLINE_CURVE_WITH_KNOTS ( 'NONE', 3,
 ( #7934, #2433, #4708, #8901 ),
 .UNSPECIFIED., .F., .F.,
 ( 4, 4 ),
 ( 0.1547128134717859205, 1.000000000000000000 ),
 .UNSPECIFIED. ) ;
#2936=AXIS2_PLACEMENT_3D ( 'NONE', #7563, #5285, #203 ) ;
#2950=EDGE_CURVE ( 'NONE', #500, #8456, #83, .T. ) ;
#2951=CARTESIAN_POINT ( 'NONE',  ( 1.105736515254441388, 3.000000000000000000, -13.50994833511691695 ) ) ;
#2953=EDGE_CURVE ( 'NONE', #10793, #3691, #3271, .T. ) ;
#2961=EDGE_CURVE ( 'NONE', #1437, #4866, #10766, .T. ) ;
#2966=ORIENTED_EDGE ( 'NONE', *, *, #6648, .T. ) ;
#2969=CARTESIAN_POINT ( 'NONE',  ( -8.922226997226788470, 3.000000000000000000, -8.158551673544387484 ) ) ;
#2973=CYLINDRICAL_SURFACE ( 'NONE', #9759, 14.25000000000000178 ) ;
#2982=ORIENTED_EDGE ( 'NONE', *, *, #13134, .T. ) ;
#2983=LINE ( 'NONE', #1816, #7970 ) ;
#2984=B_SPLINE_CURVE_WITH_KNOTS ( 'NONE', 3,
 ( #11290, #1858, #6059, #680 ),
 .UNSPECIFIED., .F., .F.,
 ( 4, 4 ),
 ( 0.000000000000000000, 0.8452273900860258760 ),
 .UNSPECIFIED. ) ;
#2990=DIRECTION ( 'NONE',  ( 0.000000000000000000, 0.000000000000000000, 1.000000000000000000 ) ) ;
#2994=CARTESIAN_POINT ( 'NONE',  ( -11.80612203322752585, 3.000000000000000000, 2.604531154829235362 ) ) ;
#2996=ORIENTED_EDGE ( 'NONE', *, *, #7201, .F. ) ;
#3003=CARTESIAN_POINT ( 'NONE',  ( -1.557181465540221188, 0.000000000000000000, 14.16466328168015743 ) ) ;
#3005=EDGE_CURVE ( 'NONE', #1142, #3822, #3941, .T. ) ;
#3010=CARTESIAN_POINT ( 'NONE',  ( 6.506507307819716424, 3.000000000000000000, -10.18987059060247269 ) ) ;
#3012=ORIENTED_EDGE ( 'NONE', *, *, #8840, .T. ) ;
#3016=CARTESIAN_POINT ( 'NONE',  ( 12.25836857253663581, 0.000000000000000000, 5.784789447945493990 ) ) ;
#3018=CARTESIAN_POINT ( 'NONE',  ( -14.08504230442587790, 3.000000000000000000, -2.161962830978695571 ) ) ;
#3019=CARTESIAN_POINT ( 'NONE',  ( 2.428572470324196431, 0.000000000000000000, 13.33579367773357127 ) ) ;
#3020=CARTESIAN_POINT ( 'NONE',  ( -10.33484986938308303, 0.000000000000000000, 8.771102293099071190 ) ) ;
#3022=CARTESIAN_POINT ( 'NONE',  ( -12.16218796965919324, 3.000000000000000000, -4.056222772158363021 ) ) ;
#3024=ORIENTED_EDGE ( 'NONE', *, *, #13248, .T. ) ;
#3025=CARTESIAN_POINT ( 'NONE',  ( -6.506507307819711095, 0.000000000000000000, 10.18987059060247624 ) ) ;
#3027=ORIENTED_EDGE ( 'NONE', *, *, #11120, .T. ) ;
#3030=FACE_OUTER_BOUND ( 'NONE', #13111, .T. ) ;
#3031=DIRECTION ( 'NONE',  ( -0.000000000000000000, -1.000000000000000000, -0.000000000000000000 ) ) ;
#3044=EDGE_CURVE ( 'NONE', #3304, #2066, #9831, .T. ) ;
#3045=LINE ( 'NONE', #2152, #2756 ) ;
#3046=EDGE_CURVE ( 'NONE', #597, #655, #820, .T. ) ;
#3049=CARTESIAN_POINT ( 'NONE',  ( 0.000000000000000000, 3.000000000000000000, 0.000000000000000000 ) ) ;
#3051=CARTESIAN_POINT ( 'NONE',  ( -7.077546079049271910, 3.000000000000000000, -10.67828022838850544 ) ) ;
#3054=DIRECTION ( 'NONE',  ( 0.000000000000000000, 0.000000000000000000, -1.000000000000000000 ) ) ;
#3061=EDGE_LOOP ( 'NONE', ( #9173, #356, #12170, #6925 ) ) ;
#3064=EDGE_CURVE ( 'NONE', #4996, #4061, #8364, .T. ) ;
#3066=CARTESIAN_POINT ( 'NONE',  ( -10.18979803820052155, 3.000000000000000000, 6.506620931068709091 ) ) ;
#3076=AXIS2_PLACEMENT_3D ( 'NONE', #1054, #6146, #2990 ) ;
#3077=CARTESIAN_POINT ( 'NONE',  ( -3.647599401157625376, 3.000000000000000000, -11.52662650599085836 ) ) ;
#3084=CARTESIAN_POINT ( 'NONE',  ( -8.922226997226891498, 3.000000000000000000, -8.158551673544284455 ) ) ;
#3087=VERTEX_POINT ( 'NONE', #5769 ) ;
#3088=DIRECTION ( 'NONE',  ( -0.000000000000000000, -1.000000000000000000, -0.000000000000000000 ) ) ;
#3089=VERTEX_POINT ( 'NONE', #12118 ) ;
#3090=CARTESIAN_POINT ( 'NONE',  ( 0.000000000000000000, 0.000000000000000000, 0.000000000000000000 ) ) ;
#3092=CARTESIAN_POINT ( 'NONE',  ( -10.18987059060247624, 0.000000000000000000, -6.506507307819711095 ) ) ;
#3094=CIRCLE ( 'NONE', #1790, 1.500000000000000222 ) ;
#3097=CARTESIAN_POINT ( 'NONE',  ( -5.170206418547658167, 0.000000000000000000, -13.27898586450066887 ) ) ;
#3110=CARTESIAN_POINT ( 'NONE',  ( -5.571313494980132397, 0.000000000000000000, 10.72979803820132005 ) ) ;
#3111=DIRECTION ( 'NONE',  ( -0.000000000000000000, -1.000000000000000000, -0.000000000000000000 ) ) ;
#3112=VECTOR ( 'NONE', #12814, 1000.000000000000000 ) ;
#3114=CARTESIAN_POINT ( 'NONE',  ( -8.430890348300632553, 3.000000000000000000, -11.48836750521723538 ) ) ;
#3115=PLANE ( 'NONE',  #10237 ) ;
#3118=ORIENTED_EDGE ( 'NONE', *, *, #4381, .T. ) ;
#3127=EDGE_CURVE ( 'NONE', #2851, #3598, #12546, .T. ) ;
#3128=CARTESIAN_POINT ( 'NONE',  ( 8.158651161643900807, 3.000000000000000000, 8.922136023539609440 ) ) ;
#3133=ORIENTED_EDGE ( 'NONE', *, *, #11069, .T. ) ;
#3136=CARTESIAN_POINT ( 'NONE',  ( -11.14709020439930676, 3.000000000000000000, -7.712570079660886257 ) ) ;
#3138=EDGE_LOOP ( 'NONE', ( #10170, #206, #8007, #10135 ) ) ;
#3144=SHAPE_DEFINITION_REPRESENTATION ( #11056, #2323 ) ;
#3145=EDGE_CURVE ( 'NONE', #205, #4996, #2853, .T. ) ;
#3147=CARTESIAN_POINT ( 'NONE',  ( 12.90250726680438476, 3.000000000000000000, 4.728042766759046778 ) ) ;
#3152=AXIS2_PLACEMENT_3D ( 'NONE', #9011, #5216, #11229 ) ;
#3155=AXIS2_PLACEMENT_3D ( 'NONE', #7761, #9960, #9886 ) ;
#3158=EDGE_LOOP ( 'NONE', ( #7301, #8563, #4698, #6630 ) ) ;
#3162=AXIS2_PLACEMENT_3D ( 'NONE', #7275, #5959, #2038 ) ;
#3163=CIRCLE ( 'NONE', #6904, 14.25000000000000178 ) ;
#3164=CARTESIAN_POINT ( 'NONE',  ( -12.14623037080100865, 0.000000000000000000, 4.072642252455982437 ) ) ;
#3166=CARTESIAN_POINT ( 'NONE',  ( 5.571313494980134173, 3.000000000000000000, -10.72979803820132005 ) ) ;
#3170=LINE ( 'NONE', #4272, #3112 ) ;
#3171=CARTESIAN_POINT ( 'NONE',  ( -12.25836857253663759, 3.000000000000000000, -5.784789447945487773 ) ) ;
#3177=ORIENTED_EDGE ( 'NONE', *, *, #9550, .T. ) ;
#3183=CARTESIAN_POINT ( 'NONE',  ( -13.33788847341978645, 0.000000000000000000, -2.414978278956336322 ) ) ;
#3185=DIRECTION ( 'NONE',  ( 0.000000000000000000, 1.000000000000000000, 0.000000000000000000 ) ) ;
#3190=CIRCLE ( 'NONE', #131, 12.08999999999737440 ) ;
#3194=CARTESIAN_POINT ( 'NONE',  ( -8.922226997226788470, 0.000000000000000000, -8.158551673544387484 ) ) ;
#3195=VERTEX_POINT ( 'NONE', #11213 ) ;
#3199=VECTOR ( 'NONE', #11440, 1000.000000000000000 ) ;
#3200=EDGE_CURVE ( 'NONE', #12067, #7218, #11004, .T. ) ;
#3212=ADVANCED_FACE ( 'NONE', ( #4949 ), #5907, .T. ) ;
#3213=ORIENTED_EDGE ( 'NONE', *, *, #1453, .F. ) ;
#3215=CARTESIAN_POINT ( 'NONE',  ( -4.072642252455976219, 3.000000000000000000, -12.14623037080101398 ) ) ;
#3224=VERTEX_POINT ( 'NONE', #7973 ) ;
#3225=DIRECTION ( 'NONE',  ( 0.000000000000000000, 1.000000000000000000, 0.000000000000000000 ) ) ;
#3226=ORIENTED_EDGE ( 'NONE', *, *, #11688, .F. ) ;
#3228=B_SPLINE_SURFACE_WITH_KNOTS ( 'NONE', 3, 1, ( 
 ( #3938, #13251 ),
 ( #12299, #2841 ),
 ( #12372, #7052 ),
 ( #8010, #13530 ) ),
 .UNSPECIFIED., .F., .F., .F.,
 ( 4, 4 ),
 ( 2, 2 ),
 ( 0.000000000000000000, 0.8452273900860258760 ),
 ( 0.000000000000000000, 1.000000000000000000 ),
 .UNSPECIFIED. ) ;
#3229=CARTESIAN_POINT ( 'NONE',  ( -13.27898586450066709, 3.000000000000000000, 5.170206418547661720 ) ) ;
#3231=CARTESIAN_POINT ( 'NONE',  ( -11.13895890373326836, 3.000000000000000000, 7.723663868796768028 ) ) ;
#3233=DIRECTION ( 'NONE',  ( 0.000000000000000000, 0.000000000000000000, 1.000000000000000000 ) ) ;
#3234=CARTESIAN_POINT ( 'NONE',  ( -10.72979803820132183, 3.000000000000000000, -5.571313494980132397 ) ) ;
#3240=B_SPLINE_CURVE_WITH_KNOTS ( 'NONE', 3,
 ( #13495, #2809, #4049, #11151 ),
 .UNSPECIFIED., .F., .F.,
 ( 4, 4 ),
 ( 0.1547128134717859205, 1.000000000000000000 ),
 .UNSPECIFIED. ) ;
#3244=DIRECTION ( 'NONE',  ( -0.000000000000000000, -1.000000000000000000, -0.000000000000000000 ) ) ;
#3255=ORIENTED_EDGE ( 'NONE', *, *, #10238, .F. ) ;
#3257=CYLINDRICAL_SURFACE ( 'NONE', #12221, 14.25000000000000355 ) ;
#3261=CARTESIAN_POINT ( 'NONE',  ( 0.000000000000000000, 0.000000000000000000, 0.000000000000000000 ) ) ;
#3270=CARTESIAN_POINT ( 'NONE',  ( 12.48034623170854474, 0.000000000000000000, 4.337627373772809491 ) ) ;
#3271=CIRCLE ( 'NONE', #5270, 14.25000000000000000 ) ;
#3278=ORIENTED_EDGE ( 'NONE', *, *, #6955, .F. ) ;
#3279=ADVANCED_FACE ( 'NONE', ( #821 ), #6990, .F. ) ;
#3280=ORIENTED_EDGE ( 'NONE', *, *, #4776, .T. ) ;
#3281=CARTESIAN_POINT ( 'NONE',  ( -2.604531154829235362, 3.000000000000000000, -11.80612203322752585 ) ) ;
#3282=EDGE_CURVE ( 'NONE', #7408, #7832, #9449, .T. ) ;
#3283=AXIS2_PLACEMENT_3D ( 'NONE', #5893, #1917, #9267 ) ;
#3284=AXIS2_PLACEMENT_3D ( 'NONE', #12904, #1120, #3448 ) ;
#3287=FACE_OUTER_BOUND ( 'NONE', #10688, .T. ) ;
#3288=B_SPLINE_CURVE_WITH_KNOTS ( 'NONE', 3,
 ( #10356, #4216, #927, #8485 ),
 .UNSPECIFIED., .F., .F.,
 ( 4, 4 ),
 ( 0.000000000000000000, 0.8452273900860258760 ),
 .UNSPECIFIED. ) ;
#3298=ORIENTED_EDGE ( 'NONE', *, *, #4056, .T. ) ;
#3300=ORIENTED_EDGE ( 'NONE', *, *, #12348, .F. ) ;
#3301=ORIENTED_EDGE ( 'NONE', *, *, #7101, .F. ) ;
#3304=VERTEX_POINT ( 'NONE', #3766 ) ;
#3305=AXIS2_PLACEMENT_3D ( 'NONE', #13148, #2748, #824 ) ;
#3306=VECTOR ( 'NONE', #2389, 1000.000000000000000 ) ;
#3308=CARTESIAN_POINT ( 'NONE',  ( 2.604531154829233586, 3.000000000000000000, 11.80612203322752585 ) ) ;
#3310=CARTESIAN_POINT ( 'NONE',  ( -11.48836750521728689, 3.000000000000000000, -8.430890348300561499 ) ) ;
#3313=FACE_OUTER_BOUND ( 'NONE', #3523, .T. ) ;
#3314=EDGE_CURVE ( 'NONE', #13127, #7310, #993, .T. ) ;
#3323=ORIENTED_EDGE ( 'NONE', *, *, #8036, .F. ) ;
#3325=CARTESIAN_POINT ( 'NONE',  ( 10.18987059060247269, 0.000000000000000000, 6.506507307819714647 ) ) ;
#3329=B_SPLINE_SURFACE_WITH_KNOTS ( 'NONE', 3, 1, ( 
 ( #13594, #3110 ),
 ( #8283, #7325 ),
 ( #11528, #1898 ),
 ( #10351, #5047 ) ),
 .UNSPECIFIED., .F., .F., .F.,
 ( 4, 4 ),
 ( 2, 2 ),
 ( 0.1547128134717859205, 1.000000000000000000 ),
 ( 0.000000000000000000, 1.000000000000000000 ),
 .UNSPECIFIED. ) ;
#3332=DIRECTION ( 'NONE',  ( 0.000000000000000000, 1.000000000000000000, 0.000000000000000000 ) ) ;
#3336=CARTESIAN_POINT ( 'NONE',  ( 10.34346111134700585, 3.000000000000000000, 8.760376775873716326 ) ) ;
#3337=B_SPLINE_SURFACE_WITH_KNOTS ( 'NONE', 3, 1, ( 
 ( #11118, #7053 ),
 ( #12158, #10974 ),
 ( #6770, #11253 ),
 ( #1687, #5879 ) ),
 .UNSPECIFIED., .F., .F., .F.,
 ( 4, 4 ),
 ( 2, 2 ),
 ( 0.000000000000000000, 0.8452273900860258760 ),
 ( 0.000000000000000000, 1.000000000000000000 ),
 .UNSPECIFIED. ) ;
#3339=CARTESIAN_POINT ( 'NONE',  ( -8.922136023539609440, 0.000000000000000000, 8.158651161643900807 ) ) ;
#3353=AXIS2_PLACEMENT_3D ( 'NONE', #8518, #11773, #12941 ) ;
#3358=EDGE_CURVE ( 'NONE', #11145, #10549, #5045, .T. ) ;
#3359=ADVANCED_FACE ( 'NONE', ( #5279 ), #8444, .F. ) ;
#3362=CARTESIAN_POINT ( 'NONE',  ( 0.000000000000000000, 3.000000000000000000, 0.000000000000000000 ) ) ;
#3371=DIRECTION ( 'NONE',  ( 0.000000000000000000, 1.000000000000000000, 0.000000000000000000 ) ) ;
#3373=ORIENTED_EDGE ( 'NONE', *, *, #3387, .T. ) ;
#3379=ADVANCED_FACE ( 'NONE', ( #11564 ), #9620, .T. ) ;
#3380=CARTESIAN_POINT ( 'NONE',  ( 31.00000000000000000, 3.000000000000000000, 3.999999998926329514 ) ) ;
#3381=DIRECTION ( 'NONE',  ( 0.000000000000000000, 0.000000000000000000, 1.000000000000000000 ) ) ;
#3384=CARTESIAN_POINT ( 'NONE',  ( -2.414978278956346092, 0.000000000000000000, 13.33788847341978467 ) ) ;
#3387=EDGE_CURVE ( 'NONE', #7832, #846, #5419, .T. ) ;
#3392=CARTESIAN_POINT ( 'NONE',  ( 0.000000000000000000, 0.000000000000000000, 0.000000000000000000 ) ) ;
#3394=ORIENTED_EDGE ( 'NONE', *, *, #6864, .F. ) ;
#3396=EDGE_LOOP ( 'NONE', ( #10299, #7048, #10491, #11825 ) ) ;
#3398=CARTESIAN_POINT ( 'NONE',  ( 0.000000000000000000, 0.000000000000000000, 0.000000000000000000 ) ) ;
#3403=DIRECTION ( 'NONE',  ( -0.000000000000000000, -1.000000000000000000, -0.000000000000000000 ) ) ;
#3405=CARTESIAN_POINT ( 'NONE',  ( 0.000000000000000000, 3.000000000000000000, 0.000000000000000000 ) ) ;
#3416=DIRECTION ( 'NONE',  ( 0.000000000000000000, 0.000000000000000000, 1.000000000000000000 ) ) ;
#3418=CARTESIAN_POINT ( 'NONE',  ( 8.158551673544282679, 0.000000000000000000, -8.922226997226884393 ) ) ;
#3421=ORIENTED_EDGE ( 'NONE', *, *, #4889, .F. ) ;
#3434=ORIENTED_EDGE ( 'NONE', *, *, #7271, .T. ) ;
#3444=VERTEX_POINT ( 'NONE', #8571 ) ;
#3448=DIRECTION ( 'NONE',  ( 0.000000000000000000, 0.000000000000000000, 1.000000000000000000 ) ) ;
#3450=CARTESIAN_POINT ( 'NONE',  ( -8.922136023539609440, 3.000000000000000000, 8.158651161643900807 ) ) ;
#3451=FACE_OUTER_BOUND ( 'NONE', #3396, .T. ) ;
#3452=ORIENTED_EDGE ( 'NONE', *, *, #1203, .T. ) ;
#3455=ADVANCED_FACE ( 'NONE', ( #4177 ), #12794, .T. ) ;
#3457=B_SPLINE_CURVE_WITH_KNOTS ( 'NONE', 3,
 ( #7627, #2526, #5551, #8647 ),
 .UNSPECIFIED., .F., .F.,
 ( 4, 4 ),
 ( 0.000000000000000000, 0.8452273900860258760 ),
 .UNSPECIFIED. ) ;
#3459=ORIENTED_EDGE ( 'NONE', *, *, #12071, .F. ) ;
#3463=CARTESIAN_POINT ( 'NONE',  ( 8.914835885878215294, 0.000000000000000000, 11.11702303352197418 ) ) ;
#3466=CARTESIAN_POINT ( 'NONE',  ( -11.48836750521723893, 0.000000000000000000, 8.430890348300625448 ) ) ;
#3482=FACE_OUTER_BOUND ( 'NONE', #112, .T. ) ;
#3484=ADVANCED_FACE ( 'NONE', ( #1617 ), #3900, .F. ) ;
#3488=ORIENTED_EDGE ( 'NONE', *, *, #4646, .T. ) ;
#3496=DIRECTION ( 'NONE',  ( -0.000000000000000000, -1.000000000000000000, -0.000000000000000000 ) ) ;
#3499=DIRECTION ( 'NONE',  ( 0.000000000000000000, 0.000000000000000000, 1.000000000000000000 ) ) ;
#3511=DIRECTION ( 'NONE',  ( 0.000000000000000000, 0.000000000000000000, -1.000000000000000000 ) ) ;
#3513=EDGE_CURVE ( 'NONE', #11907, #12112, #7865, .T. ) ;
#3523=EDGE_LOOP ( 'NONE', ( #12464, #10452, #1777, #9402 ) ) ;
#3532=CARTESIAN_POINT ( 'NONE',  ( -14.16466328168010769, 0.000000000000000000, -1.557181465540673271 ) ) ;
#3534=CIRCLE ( 'NONE', #686, 14.24999999999999822 ) ;
#3539=CARTESIAN_POINT ( 'NONE',  ( 10.18979803820051622, 0.000000000000000000, -6.506620931068703761 ) ) ;
#3541=ORIENTED_EDGE ( 'NONE', *, *, #7621, .T. ) ;
#3542=CARTESIAN_POINT ( 'NONE',  ( 5.571433138827823761, 3.000000000000000000, 10.72973591378220704 ) ) ;
#3545=CARTESIAN_POINT ( 'NONE',  ( -8.922226997226788470, 3.000000000000000000, -8.158551673544387484 ) ) ;
#3547=LINE ( 'NONE', #5418, #4415 ) ;
#3550=EDGE_CURVE ( 'NONE', #7698, #11304, #6370, .T. ) ;
#3556=EDGE_LOOP ( 'NONE', ( #3226, #5503, #9259, #1666 ) ) ;
#3558=CARTESIAN_POINT ( 'NONE',  ( 0.000000000000000000, 3.000000000000000000, 0.000000000000000000 ) ) ;
#3559=EDGE_LOOP ( 'NONE', ( #1967, #12488, #7497, #5799 ) ) ;
#3568=FACE_BOUND ( 'NONE', #12002, .T. ) ;
#3587=CARTESIAN_POINT ( 'NONE',  ( 0.5400000000008007284, 0.000000000000000000, 12.07793442604883793 ) ) ;
#3590=CARTESIAN_POINT ( 'NONE',  ( 0.000000000000000000, 0.000000000000000000, 0.000000000000000000 ) ) ;
#3591=EDGE_LOOP ( 'NONE', ( #3024, #5472, #1836, #5702 ) ) ;
#3597=CIRCLE ( 'NONE', #2074, 1.500000000000000222 ) ;
#3598=VERTEX_POINT ( 'NONE', #9682 ) ;
#3600=CARTESIAN_POINT ( 'NONE',  ( 4.056222772158357692, 3.000000000000000000, -12.16218796965919680 ) ) ;
#3603=B_SPLINE_CURVE_WITH_KNOTS ( 'NONE', 3,
 ( #10654, #1482, #246, #5533 ),
 .UNSPECIFIED., .F., .F.,
 ( 4, 4 ),
 ( 0.1547128134717859205, 1.000000000000000000 ),
 .UNSPECIFIED. ) ;
#3605=AXIS2_PLACEMENT_3D ( 'NONE', #3757, #7885, #5686 ) ;
#3608=CARTESIAN_POINT ( 'NONE',  ( -10.18987059060247624, 3.000000000000000000, -6.506507307819711095 ) ) ;
#3615=VECTOR ( 'NONE', #4496, 1000.000000000000000 ) ;
#3616=ORIENTED_EDGE ( 'NONE', *, *, #8932, .T. ) ;
#3618=CYLINDRICAL_SURFACE ( 'NONE', #4498, 12.08999999999737440 ) ;
#3621=CARTESIAN_POINT ( 'NONE',  ( 11.48836750521724070, 0.000000000000000000, -8.430890348300621895 ) ) ;
#3628=ORIENTED_EDGE ( 'NONE', *, *, #4378, .F. ) ;
#3630=ORIENTED_EDGE ( 'NONE', *, *, #10402, .F. ) ;
#3633=EDGE_CURVE ( 'NONE', #7408, #6519, #9244, .T. ) ;
#3646=ORIENTED_EDGE ( 'NONE', *, *, #2669, .F. ) ;
#3647=CARTESIAN_POINT ( 'NONE',  ( 1.836970198721030181E-16, 0.000000000000000000, 1.500000000000000222 ) ) ;
#3654=FACE_OUTER_BOUND ( 'NONE', #12458, .T. ) ;
#3655=ORIENTED_EDGE ( 'NONE', *, *, #10658, .T. ) ;
#3659=EDGE_CURVE ( 'NONE', #5441, #10694, #12554, .T. ) ;
#3661=ORIENTED_EDGE ( 'NONE', *, *, #6558, .T. ) ;
#3673=CARTESIAN_POINT ( 'NONE',  ( 0.000000000000000000, 3.000000000000000000, 0.000000000000000000 ) ) ;
#3674=ORIENTED_EDGE ( 'NONE', *, *, #12150, .T. ) ;
#3676=B_SPLINE_SURFACE_WITH_KNOTS ( 'NONE', 3, 1, ( 
 ( #3084, #9367 ),
 ( #13429, #4121 ),
 ( #3985, #12541 ),
 ( #8181, #11495 ) ),
 .UNSPECIFIED., .F., .F., .F.,
 ( 4, 4 ),
 ( 2, 2 ),
 ( 0.1547128134717859205, 1.000000000000000000 ),
 ( 0.000000000000000000, 1.000000000000000000 ),
 .UNSPECIFIED. ) ;
#3681=CARTESIAN_POINT ( 'NONE',  ( 31.00000000000000000, 3.000000000000000000, 3.999999998926329514 ) ) ;
#3682=CARTESIAN_POINT ( 'NONE',  ( -2.161962830978783057, 3.000000000000000000, -14.08504230442586369 ) ) ;
#3688=ORIENTED_EDGE ( 'NONE', *, *, #7105, .T. ) ;
#3691=VERTEX_POINT ( 'NONE', #12374 ) ;
#3694=EDGE_CURVE ( 'NONE', #8654, #5917, #5278, .T. ) ;
#3697=ADVANCED_FACE ( 'NONE', ( #8341 ), #2843, .T. ) ;
#3698=FACE_OUTER_BOUND ( 'NONE', #9826, .T. ) ;
#3699=CARTESIAN_POINT ( 'NONE',  ( -2.604531154829235362, 3.000000000000000000, -11.80612203322752585 ) ) ;
#3703=EDGE_CURVE ( 'NONE', #1162, #2665, #8683, .T. ) ;
#3708=CARTESIAN_POINT ( 'NONE',  ( -7.712570079660889810, 0.000000000000000000, 11.14709020439930320 ) ) ;
#3713=CARTESIAN_POINT ( 'NONE',  ( -11.52662650599092409, 3.000000000000000000, 3.647599401157420651 ) ) ;
#3715=CARTESIAN_POINT ( 'NONE',  ( 0.000000000000000000, 0.000000000000000000, 0.000000000000000000 ) ) ;
#3719=CARTESIAN_POINT ( 'NONE',  ( -0.7901945867173586491, 0.000000000000000000, -12.78643498603818074 ) ) ;
#3720=VERTEX_POINT ( 'NONE', #6022 ) ;
#3722=EDGE_CURVE ( 'NONE', #9128, #6683, #6597, .T. ) ;
#3737=CARTESIAN_POINT ( 'NONE',  ( 0.000000000000000000, 0.000000000000000000, 0.000000000000000000 ) ) ;
#3744=B_SPLINE_CURVE_WITH_KNOTS ( 'NONE', 3,
 ( #4877, #2812, #9472, #9214 ),
 .UNSPECIFIED., .F., .F.,
 ( 4, 4 ),
 ( 0.000000000000000000, 0.8452273900860258760 ),
 .UNSPECIFIED. ) ;
#3748=CARTESIAN_POINT ( 'NONE',  ( 6.506620931068708202, 3.000000000000000000, 10.18979803820052155 ) ) ;
#3753=DIRECTION ( 'NONE',  ( -0.000000000000000000, -1.000000000000000000, -0.000000000000000000 ) ) ;
#3755=CARTESIAN_POINT ( 'NONE',  ( 0.000000000000000000, 3.000000000000000000, -1.500000000000000222 ) ) ;
#3757=CARTESIAN_POINT ( 'NONE',  ( 0.000000000000000000, 3.000000000000000000, 0.000000000000000000 ) ) ;
#3758=CARTESIAN_POINT ( 'NONE',  ( -10.72973591378220348, 3.000000000000000000, 5.571433138827830867 ) ) ;
#3762=VECTOR ( 'NONE', #3403, 1000.000000000000000 ) ;
#3766=CARTESIAN_POINT ( 'NONE',  ( -5.733772933379472470, 3.000000000000000000, 13.04554897075799502 ) ) ;
#3775=DIRECTION ( 'NONE',  ( -0.000000000000000000, -1.000000000000000000, -0.000000000000000000 ) ) ;
#3776=ORIENTED_EDGE ( 'NONE', *, *, #2615, .T. ) ;
#3778=VECTOR ( 'NONE', #60, 1000.000000000000000 ) ;
#3781=AXIS2_PLACEMENT_3D ( 'NONE', #475, #3496, #8732 ) ;
#3793=CARTESIAN_POINT ( 'NONE',  ( -13.04554897075799680, 0.000000000000000000, -5.733772933379471581 ) ) ;
#3797=EDGE_LOOP ( 'NONE', ( #13188, #12752, #9385, #10487 ) ) ;
#3799=VERTEX_POINT ( 'NONE', #10757 ) ;
#3805=AXIS2_PLACEMENT_3D ( 'NONE', #1045, #10339, #5241 ) ;
#3807=EDGE_CURVE ( 'NONE', #9307, #1347, #5941, .T. ) ;
#3813=CARTESIAN_POINT ( 'NONE',  ( 0.000000000000000000, 3.000000000000000000, 0.000000000000000000 ) ) ;
#3816=B_SPLINE_CURVE_WITH_KNOTS ( 'NONE', 3,
 ( #8064, #951, #5859, #7354 ),
 .UNSPECIFIED., .F., .F.,
 ( 4, 4 ),
 ( 0.1547128134717859205, 1.000000000000000000 ),
 .UNSPECIFIED. ) ;
#3821=CIRCLE ( 'NONE', #10860, 12.08999999999737440 ) ;
#3822=VERTEX_POINT ( 'NONE', #2289 ) ;
#3828=VECTOR ( 'NONE', #1372, 1000.000000000000000 ) ;
#3833=CARTESIAN_POINT ( 'NONE',  ( 10.69794375946289655, 0.000000000000000000, 7.065816209474157006 ) ) ;
#3843=EDGE_LOOP ( 'NONE', ( #6191, #414, #12556, #2902 ) ) ;
#3845=CARTESIAN_POINT ( 'NONE',  ( -2.428572470324203980, 0.000000000000000000, -13.33579367773357482 ) ) ;
#3847=CIRCLE ( 'NONE', #9349, 14.24999999999999822 ) ;
#3848=LINE ( 'NONE', #8048, #41 ) ;
#3853=VERTEX_POINT ( 'NONE', #11657 ) ;
#3858=ORIENTED_EDGE ( 'NONE', *, *, #8687, .T. ) ;
#3862=DIRECTION ( 'NONE',  ( -0.000000000000000000, -1.000000000000000000, -0.000000000000000000 ) ) ;
#3864=CARTESIAN_POINT ( 'NONE',  ( -14.16466328168009881, 3.000000000000000000, 1.557181465540760534 ) ) ;
#3878=DIRECTION ( 'NONE',  ( 0.000000000000000000, 1.000000000000000000, 0.000000000000000000 ) ) ;
#3891=LINE ( 'NONE', #8296, #7360 ) ;
#3900=B_SPLINE_SURFACE_WITH_KNOTS ( 'NONE', 3, 1, ( 
 ( #4781, #719 ),
 ( #10078, #8968 ),
 ( #6582, #9115 ),
 ( #13179, #6840 ) ),
 .UNSPECIFIED., .F., .F., .F.,
 ( 4, 4 ),
 ( 2, 2 ),
 ( 0.000000000000000000, 0.8452273900860258760 ),
 ( 0.000000000000000000, 1.000000000000000000 ),
 .UNSPECIFIED. ) ;
#3907=FACE_OUTER_BOUND ( 'NONE', #8653, .T. ) ;
#3912=DIRECTION ( 'NONE',  ( -0.000000000000000000, -1.000000000000000000, -0.000000000000000000 ) ) ;
#3914=ORIENTED_EDGE ( 'NONE', *, *, #11390, .T. ) ;
#3915=CARTESIAN_POINT ( 'NONE',  ( 12.48034623170854474, 0.000000000000000000, 4.337627373772809491 ) ) ;
#3920=ORIENTED_EDGE ( 'NONE', *, *, #2613, .F. ) ;
#3932=VERTEX_POINT ( 'NONE', #7458 ) ;
#3936=ADVANCED_FACE ( 'NONE', ( #5792 ), #9852, .F. ) ;
#3938=CARTESIAN_POINT ( 'NONE',  ( 11.11702303352191912, 3.000000000000000000, -8.914835885878277466 ) ) ;
#3939=CARTESIAN_POINT ( 'NONE',  ( 0.000000000000000000, 3.000000000000000000, 0.000000000000000000 ) ) ;
#3941=CIRCLE ( 'NONE', #7258, 12.08999999999737440 ) ;
#3947=DIRECTION ( 'NONE',  ( -0.000000000000000000, -1.000000000000000000, -0.000000000000000000 ) ) ;
#3949=ORIENTED_EDGE ( 'NONE', *, *, #4060, .T. ) ;
#3956=EDGE_CURVE ( 'NONE', #10361, #1111, #11449, .T. ) ;
#3959=ADVANCED_FACE ( 'NONE', ( #7721 ), #7107, .F. ) ;
#3961=DIRECTION ( 'NONE',  ( 0.000000000000000000, 1.000000000000000000, 0.000000000000000000 ) ) ;
#3968=CARTESIAN_POINT ( 'NONE',  ( 12.25836857253663581, 0.000000000000000000, 5.784789447945493990 ) ) ;
#3970=EDGE_CURVE ( 'NONE', #8320, #13244, #8793, .T. ) ;
#3979=CARTESIAN_POINT ( 'NONE',  ( -11.11702303352191734, 0.000000000000000000, 8.914835885878279242 ) ) ;
#3985=CARTESIAN_POINT ( 'NONE',  ( -10.34346111134701118, 3.000000000000000000, -8.760376775873707444 ) ) ;
#3992=CARTESIAN_POINT ( 'NONE',  ( -10.18987059060247624, 0.000000000000000000, -6.506507307819711095 ) ) ;
#3993=CARTESIAN_POINT ( 'NONE',  ( -7.065816209474154341, 0.000000000000000000, 10.69794375946289833 ) ) ;
#3995=FACE_OUTER_BOUND ( 'NONE', #4775, .T. ) ;
#3996=LINE ( 'NONE', #2900, #2457 ) ;
#4000=CARTESIAN_POINT ( 'NONE',  ( 10.18979803820051622, 3.000000000000000000, -6.506620931068703761 ) ) ;
#4008=ORIENTED_EDGE ( 'NONE', *, *, #12061, .T. ) ;
#4012=CARTESIAN_POINT ( 'NONE',  ( 10.18979803820051622, 3.000000000000000000, -6.506620931068703761 ) ) ;
#4014=CIRCLE ( 'NONE', #4449, 12.08999999999737263 ) ;
#4020=LINE ( 'NONE', #4092, #1103 ) ;
#4022=B_SPLINE_CURVE_WITH_KNOTS ( 'NONE', 3,
 ( #4041, #6110, #1774, #8105 ),
 .UNSPECIFIED., .F., .F.,
 ( 4, 4 ),
 ( 0.000000000000000000, 0.8452273900860258760 ),
 .UNSPECIFIED. ) ;
#4024=CARTESIAN_POINT ( 'NONE',  ( 5.170206418547656391, 0.000000000000000000, 13.27898586450067064 ) ) ;
#4036=AXIS2_PLACEMENT_3D ( 'NONE', #1793, #1930, #5987 ) ;
#4041=CARTESIAN_POINT ( 'NONE',  ( 13.04554897075798081, 3.000000000000000000, -5.733772933379503556 ) ) ;
#4049=CARTESIAN_POINT ( 'NONE',  ( 1.119409668803368119, 3.000000000000000000, 13.50845331674225847 ) ) ;
#4050=CARTESIAN_POINT ( 'NONE',  ( 4.056222772158357692, 0.000000000000000000, -12.16218796965919680 ) ) ;
#4056=EDGE_CURVE ( 'NONE', #7832, #6591, #13576, .T. ) ;
#4058=VERTEX_POINT ( 'NONE', #8069 ) ;
#4060=EDGE_CURVE ( 'NONE', #4189, #9400, #12115, .T. ) ;
#4061=VERTEX_POINT ( 'NONE', #7241 ) ;
#4062=DIRECTION ( 'NONE',  ( 0.000000000000000000, 0.000000000000000000, -1.000000000000000000 ) ) ;
#4073=DIRECTION ( 'NONE',  ( -0.000000000000000000, -1.000000000000000000, -0.000000000000000000 ) ) ;
#4074=CARTESIAN_POINT ( 'NONE',  ( -10.72979803820132183, 0.000000000000000000, -5.571313494980132397 ) ) ;
#4077=CARTESIAN_POINT ( 'NONE',  ( 0.000000000000000000, 0.000000000000000000, 0.000000000000000000 ) ) ;
#4079=EDGE_LOOP ( 'NONE', ( #7404, #2460 ) ) ;
#4081=CARTESIAN_POINT ( 'NONE',  ( -8.158651161643904359, 0.000000000000000000, -8.922136023539605887 ) ) ;
#4083=VERTEX_POINT ( 'NONE', #12811 ) ;
#4089=FACE_OUTER_BOUND ( 'NONE', #6208, .T. ) ;
#4090=CARTESIAN_POINT ( 'NONE',  ( 0.000000000000000000, 0.000000000000000000, 0.000000000000000000 ) ) ;
#4092=CARTESIAN_POINT ( 'NONE',  ( -5.170206418547658167, 3.000000000000000000, -13.27898586450066887 ) ) ;
#4096=DIRECTION ( 'NONE',  ( -0.000000000000000000, -1.000000000000000000, -0.000000000000000000 ) ) ;
#4105=CARTESIAN_POINT ( 'NONE',  ( 0.000000000000000000, 0.000000000000000000, 0.000000000000000000 ) ) ;
#4107=CARTESIAN_POINT ( 'NONE',  ( -13.50994833511691340, 3.000000000000000000, -1.105736515254444052 ) ) ;
#4108=EDGE_LOOP ( 'NONE', ( #13586, #6102, #4548, #10588 ) ) ;
#4109=ADVANCED_FACE ( 'NONE', ( #1169 ), #8589, .F. ) ;
#4114=ADVANCED_FACE ( 'NONE', ( #3287 ), #6112, .F. ) ;
#4121=CARTESIAN_POINT ( 'NONE',  ( -9.600126836553261711, 0.000000000000000000, -8.482622935103767858 ) ) ;
#4123=ORIENTED_EDGE ( 'NONE', *, *, #11037, .T. ) ;
#4130=EDGE_CURVE ( 'NONE', #9203, #5441, #8811, .T. ) ;
#4131=CARTESIAN_POINT ( 'NONE',  ( 5.733772933379453818, 3.000000000000000000, 13.04554897075800568 ) ) ;
#4138=CARTESIAN_POINT ( 'NONE',  ( 0.000000000000000000, 0.000000000000000000, 0.000000000000000000 ) ) ;
#4140=ORIENTED_EDGE ( 'NONE', *, *, #10526, .T. ) ;
#4141=DIRECTION ( 'NONE',  ( -0.000000000000000000, -1.000000000000000000, -0.000000000000000000 ) ) ;
#4148=CARTESIAN_POINT ( 'NONE',  ( 11.11702303352196708, 0.000000000000000000, 8.914835885878218846 ) ) ;
#4154=ORIENTED_EDGE ( 'NONE', *, *, #6084, .F. ) ;
#4156=ORIENTED_EDGE ( 'NONE', *, *, #13079, .F. ) ;
#4160=EDGE_CURVE ( 'NONE', #13268, #5502, #6821, .T. ) ;
#4164=LINE ( 'NONE', #7213, #9079 ) ;
#4165=CARTESIAN_POINT ( 'NONE',  ( -11.80615107470192804, 0.000000000000000000, -2.604399508764160487 ) ) ;
#4169=ORIENTED_EDGE ( 'NONE', *, *, #5148, .T. ) ;
#4176=VECTOR ( 'NONE', #8282, 1000.000000000000000 ) ;
#4177=FACE_OUTER_BOUND ( 'NONE', #4608, .T. ) ;
#4185=ORIENTED_EDGE ( 'NONE', *, *, #6647, .T. ) ;
#4188=DIRECTION ( 'NONE',  ( -0.000000000000000000, -1.000000000000000000, -0.000000000000000000 ) ) ;
#4189=VERTEX_POINT ( 'NONE', #11583 ) ;
#4191=FILL_AREA_STYLE_COLOUR ( '', #2540 ) ;
#4194=CARTESIAN_POINT ( 'NONE',  ( 5.784789447945496654, 3.000000000000000000, -12.25836857253663581 ) ) ;
#4204=DIRECTION ( 'NONE',  ( 0.000000000000000000, 0.000000000000000000, -1.000000000000000000 ) ) ;
#4216=CARTESIAN_POINT ( 'NONE',  ( -2.428572470324203980, 0.000000000000000000, -13.33579367773357482 ) ) ;
#4220=EDGE_CURVE ( 'NONE', #13138, #6731, #11002, .T. ) ;
#4223=ORIENTED_EDGE ( 'NONE', *, *, #1134, .F. ) ;
#4228=CIRCLE ( 'NONE', #11934, 12.08999999999737440 ) ;
#4235=AXIS2_PLACEMENT_3D ( 'NONE', #787, #1746, #643 ) ;
#4238=AXIS2_PLACEMENT_3D ( 'NONE', #6225, #862, #5053 ) ;
#4241=B_SPLINE_SURFACE_WITH_KNOTS ( 'NONE', 3, 1, ( 
 ( #10181, #5015 ),
 ( #13423, #8177 ),
 ( #12480, #12409 ),
 ( #3018, #7225 ) ),
 .UNSPECIFIED., .F., .F., .F.,
 ( 4, 4 ),
 ( 2, 2 ),
 ( 0.1547128134717859205, 1.000000000000000000 ),
 ( 0.000000000000000000, 1.000000000000000000 ),
 .UNSPECIFIED. ) ;
#4244=CARTESIAN_POINT ( 'NONE',  ( -10.18987059060247624, 3.000000000000000000, -6.506507307819711095 ) ) ;
#4248=AXIS2_PLACEMENT_3D ( 'NONE', #8669, #355, #1180 ) ;
#4249=CARTESIAN_POINT ( 'NONE',  ( 0.000000000000000000, 0.000000000000000000, 0.000000000000000000 ) ) ;
#4256=CARTESIAN_POINT ( 'NONE',  ( 4.072642252455978884, 0.000000000000000000, 12.14623037080101042 ) ) ;
#4269=DIRECTION ( 'NONE',  ( 0.000000000000000000, 1.000000000000000000, 0.000000000000000000 ) ) ;
#4272=CARTESIAN_POINT ( 'NONE',  ( 2.604531154829233586, 3.000000000000000000, 11.80612203322752585 ) ) ;
#4274=VERTEX_POINT ( 'NONE', #12120 ) ;
#4277=VERTEX_POINT ( 'NONE', #1656 ) ;
#4281=FACE_OUTER_BOUND ( 'NONE', #5664, .T. ) ;
#4282=VERTEX_POINT ( 'NONE', #617 ) ;
#4283=CARTESIAN_POINT ( 'NONE',  ( 3.647599401157688437, 3.000000000000000000, 11.52662650599083882 ) ) ;
#4284=CARTESIAN_POINT ( 'NONE',  ( 10.18987059060247269, 3.000000000000000000, 6.506507307819714647 ) ) ;
#4288=CARTESIAN_POINT ( 'NONE',  ( 13.27898586450067242, 3.000000000000000000, -5.170206418547655502 ) ) ;
#4290=VECTOR ( 'NONE', #12444, 1000.000000000000000 ) ;
#4296=CARTESIAN_POINT ( 'NONE',  ( 12.25282671965375592, 0.000000000000000000, -5.797378255456012930 ) ) ;
#4300=EDGE_LOOP ( 'NONE', ( #9691, #546, #267, #980 ) ) ;
#4307=CARTESIAN_POINT ( 'NONE',  ( 0.000000000000000000, 3.000000000000000000, 0.000000000000000000 ) ) ;
#4309=CARTESIAN_POINT ( 'NONE',  ( -11.13895890373326836, 3.000000000000000000, 7.723663868796768028 ) ) ;
#4311=LINE ( 'NONE', #12782, #5738 ) ;
#4313=EDGE_CURVE ( 'NONE', #544, #843, #12944, .T. ) ;
#4314=DIRECTION ( 'NONE',  ( 0.000000000000000000, 0.000000000000000000, 1.000000000000000000 ) ) ;
#4320=CARTESIAN_POINT ( 'NONE',  ( -12.07793442604884682, 3.000000000000000000, 0.5400000000005513723 ) ) ;
#4323=EDGE_CURVE ( 'NONE', #11264, #4866, #13212, .T. ) ;
#4337=EDGE_CURVE ( 'NONE', #544, #11807, #3094, .T. ) ;
#4339=( LENGTH_UNIT ( ) NAMED_UNIT ( * ) SI_UNIT ( .MILLI., .METRE. ) );
#4342=DIRECTION ( 'NONE',  ( -0.000000000000000000, -1.000000000000000000, -0.000000000000000000 ) ) ;
#4344=CARTESIAN_POINT ( 'NONE',  ( -11.52662650599092409, 3.000000000000000000, 3.647599401157420651 ) ) ;
#4346=ORIENTED_EDGE ( 'NONE', *, *, #1201, .F. ) ;
#4350=ORIENTED_EDGE ( 'NONE', *, *, #7532, .T. ) ;
#4352=ORIENTED_EDGE ( 'NONE', *, *, #8764, .T. ) ;
#4353=LINE ( 'NONE', #7519, #6928 ) ;
#4358=CARTESIAN_POINT ( 'NONE',  ( 2.414978278956333213, 3.000000000000000000, -13.33788847341978645 ) ) ;
#4361=ORIENTED_EDGE ( 'NONE', *, *, #8708, .F. ) ;
#4362=CARTESIAN_POINT ( 'NONE',  ( -3.647470871583628593, 0.000000000000000000, 11.52666717836884125 ) ) ;
#4363=EDGE_LOOP ( 'NONE', ( #12189, #3255, #5453, #9314 ) ) ;
#4364=EDGE_LOOP ( 'NONE', ( #5842, #6372, #10186, #10436 ) ) ;
#4365=EDGE_CURVE ( 'NONE', #7906, #6233, #6538, .T. ) ;
#4366=ORIENTED_EDGE ( 'NONE', *, *, #4706, .F. ) ;
#4368=CARTESIAN_POINT ( 'NONE',  ( -1.557181465540221188, 0.000000000000000000, 14.16466328168015743 ) ) ;
#4369=CARTESIAN_POINT ( 'NONE',  ( 11.14709020439929787, 0.000000000000000000, 7.712570079660892475 ) ) ;
#4372=CARTESIAN_POINT ( 'NONE',  ( -2.161962830978702677, 3.000000000000000000, 14.08504230442587435 ) ) ;
#4373=VECTOR ( 'NONE', #4892, 1000.000000000000000 ) ;
#4377=FACE_OUTER_BOUND ( 'NONE', #7770, .T. ) ;
#4378=EDGE_CURVE ( 'NONE', #1810, #1061, #8789, .T. ) ;
#4381=EDGE_CURVE ( 'NONE', #2083, #1162, #9692, .T. ) ;
#4388=CARTESIAN_POINT ( 'NONE',  ( 5.170206418547656391, 0.000000000000000000, 13.27898586450067064 ) ) ;
#4389=ADVANCED_FACE ( 'NONE', ( #10256 ), #9210, .T. ) ;
#4397=ADVANCED_FACE ( 'NONE', ( #3907 ), #11620, .F. ) ;
#4400=DIRECTION ( 'NONE',  ( 0.000000000000000000, 0.000000000000000000, 1.000000000000000000 ) ) ;
#4405=CARTESIAN_POINT ( 'NONE',  ( -12.56087513340552242, 0.000000000000000000, 2.568302020731519253 ) ) ;
#4407=ORIENTED_EDGE ( 'NONE', *, *, #8491, .F. ) ;
#4408=DIRECTION ( 'NONE',  ( -0.000000000000000000, -1.000000000000000000, -0.000000000000000000 ) ) ;
#4414=ORIENTED_EDGE ( 'NONE', *, *, #12477, .T. ) ;
#4415=VECTOR ( 'NONE', #10863, 1000.000000000000000 ) ;
#4438=CARTESIAN_POINT ( 'NONE',  ( -2.604531154829235362, 0.000000000000000000, -11.80612203322752585 ) ) ;
#4442=VERTEX_POINT ( 'NONE', #886 ) ;
#4444=B_SPLINE_SURFACE_WITH_KNOTS ( 'NONE', 3, 1, ( 
 ( #10884, #1449 ),
 ( #5639, #9836 ),
 ( #408, #4606 ),
 ( #9549, #9153 ) ),
 .UNSPECIFIED., .F., .F., .F.,
 ( 4, 4 ),
 ( 2, 2 ),
 ( 0.1547128134717859205, 1.000000000000000000 ),
 ( 0.000000000000000000, 1.000000000000000000 ),
 .UNSPECIFIED. ) ;
#4449=AXIS2_PLACEMENT_3D ( 'NONE', #11173, #5933, #1534 ) ;
#4451=DIRECTION ( 'NONE',  ( 0.000000000000000000, 1.000000000000000000, 0.000000000000000000 ) ) ;
#4452=EDGE_CURVE ( 'NONE', #5502, #6360, #3240, .T. ) ;
#4453=CARTESIAN_POINT ( 'NONE',  ( -13.04554897075799680, 3.000000000000000000, -5.733772933379471581 ) ) ;
#4455=CARTESIAN_POINT ( 'NONE',  ( 1.105736515254441388, 0.000000000000000000, -13.50994833511691695 ) ) ;
#4461=DIRECTION ( 'NONE',  ( 0.000000000000000000, 1.000000000000000000, 0.000000000000000000 ) ) ;
#4462=AXIS2_PLACEMENT_3D ( 'NONE', #4307, #7818, #1011 ) ;
#4468=CARTESIAN_POINT ( 'NONE',  ( 5.708888906988906164, 0.000000000000000000, -11.46847481510586775 ) ) ;
#4469=B_SPLINE_CURVE_WITH_KNOTS ( 'NONE', 3,
 ( #2449, #12793, #8569, #3339 ),
 .UNSPECIFIED., .F., .F.,
 ( 4, 4 ),
 ( 0.000000000000000000, 0.8452273900860258760 ),
 .UNSPECIFIED. ) ;
#4478=ORIENTED_EDGE ( 'NONE', *, *, #3005, .F. ) ;
#4479=ADVANCED_FACE ( 'NONE', ( #7019 ), #4241, .F. ) ;
#4481=EDGE_LOOP ( 'NONE', ( #6117, #10887, #13039, #3776 ) ) ;
#4482=EDGE_CURVE ( 'NONE', #13298, #12936, #4857, .T. ) ;
#4483=ORIENTED_EDGE ( 'NONE', *, *, #3358, .F. ) ;
#4487=AXIS2_PLACEMENT_3D ( 'NONE', #11642, #10682, #6398 ) ;
#4492=EDGE_CURVE ( 'NONE', #7043, #11145, #3848, .T. ) ;
#4495=CARTESIAN_POINT ( 'NONE',  ( -10.33484986938308303, 3.000000000000000000, 8.771102293099071190 ) ) ;
#4496=DIRECTION ( 'NONE',  ( -1.000000000000000000, 0.000000000000000000, 1.370446048119726253E-16 ) ) ;
#4498=AXIS2_PLACEMENT_3D ( 'NONE', #7817, #7880, #4728 ) ;
#4500=VECTOR ( 'NONE', #13150, 1000.000000000000000 ) ;
#4504=ORIENTED_EDGE ( 'NONE', *, *, #9144, .T. ) ;
#4506=VECTOR ( 'NONE', #9805, 1000.000000000000000 ) ;
#4514=CARTESIAN_POINT ( 'NONE',  ( 0.000000000000000000, 3.000000000000000000, 0.000000000000000000 ) ) ;
#4518=ORIENTED_EDGE ( 'NONE', *, *, #1256, .T. ) ;
#4523=( GEOMETRIC_REPRESENTATION_CONTEXT ( 3 ) GLOBAL_UNCERTAINTY_ASSIGNED_CONTEXT ( ( #5578 ) ) GLOBAL_UNIT_ASSIGNED_CONTEXT ( ( #4339, #12686, #1098 ) ) REPRESENTATION_CONTEXT ( 'NONE', 'WORKASPACE' ) );
#4530=ORIENTED_EDGE ( 'NONE', *, *, #6673, .F. ) ;
#4536=EDGE_CURVE ( 'NONE', #6360, #9461, #3534, .T. ) ;
#4542=FACE_OUTER_BOUND ( 'NONE', #9778, .T. ) ;
#4548=ORIENTED_EDGE ( 'NONE', *, *, #9812, .F. ) ;
#4553=ORIENTED_EDGE ( 'NONE', *, *, #6010, .T. ) ;
#4556=EDGE_CURVE ( 'NONE', #9203, #10050, #10727, .T. ) ;
#4557=CARTESIAN_POINT ( 'NONE',  ( 2.161962830978694683, 3.000000000000000000, -14.08504230442587790 ) ) ;
#4561=CARTESIAN_POINT ( 'NONE',  ( 8.922136023539611216, 3.000000000000000000, -8.158651161643899030 ) ) ;
#4563=ORIENTED_EDGE ( 'NONE', *, *, #8504, .T. ) ;
#4569=ORIENTED_EDGE ( 'NONE', *, *, #11808, .F. ) ;
#4570=LINE ( 'NONE', #6706, #2076 ) ;
#4571=CARTESIAN_POINT ( 'NONE',  ( 5.170206418547588001, 0.000000000000000000, -13.27898586450069907 ) ) ;
#4572=EDGE_CURVE ( 'NONE', #4442, #13298, #2057, .T. ) ;
#4574=FACE_OUTER_BOUND ( 'NONE', #6923, .T. ) ;
#4578=ORIENTED_EDGE ( 'NONE', *, *, #1274, .F. ) ;
#4590=DIRECTION ( 'NONE',  ( 0.000000000000000000, 0.000000000000000000, 1.000000000000000000 ) ) ;
#4592=CARTESIAN_POINT ( 'NONE',  ( 31.00000000000000000, 3.000000000000000000, -1.073670993220974656E-09 ) ) ;
#4593=CARTESIAN_POINT ( 'NONE',  ( 8.771102293099069414, 0.000000000000000000, 10.33484986938308303 ) ) ;
#4599=ORIENTED_EDGE ( 'NONE', *, *, #2799, .T. ) ;
#4602=AXIS2_PLACEMENT_3D ( 'NONE', #4249, #1986, #8309 ) ;
#4604=CARTESIAN_POINT ( 'NONE',  ( -11.11702303352197063, 0.000000000000000000, -8.914835885878215294 ) ) ;
#4606=CARTESIAN_POINT ( 'NONE',  ( 8.760376775873721655, 0.000000000000000000, -10.34346111134700585 ) ) ;
#4608=EDGE_LOOP ( 'NONE', ( #612, #10566, #3646, #7173 ) ) ;
#4609=CARTESIAN_POINT ( 'NONE',  ( -5.797378255456022700, 3.000000000000000000, -12.25282671965375592 ) ) ;
#4610=EDGE_LOOP ( 'NONE', ( #3914, #6530, #4530, #2350 ) ) ;
#4611=VECTOR ( 'NONE', #8903, 1000.000000000000000 ) ;
#4614=ORIENTED_EDGE ( 'NONE', *, *, #3200, .F. ) ;
#4634=CARTESIAN_POINT ( 'NONE',  ( 5.170206418547588001, 3.000000000000000000, -13.27898586450069907 ) ) ;
#4641=CARTESIAN_POINT ( 'NONE',  ( 5.731782959214990036, 3.000000000000000000, 11.46814821560793618 ) ) ;
#4646=EDGE_CURVE ( 'NONE', #8355, #3822, #4732, .T. ) ;
#4650=EDGE_LOOP ( 'NONE', ( #6464, #10617, #57, #4504 ) ) ;
#4659=VECTOR ( 'NONE', #3912, 1000.000000000000000 ) ;
#4660=CYLINDRICAL_SURFACE ( 'NONE', #2295, 12.08999999999737263 ) ;
#4661=CARTESIAN_POINT ( 'NONE',  ( 5.170206418547656391, 3.000000000000000000, 13.27898586450067064 ) ) ;
#4662=VERTEX_POINT ( 'NONE', #3681 ) ;
#4664=ORIENTED_EDGE ( 'NONE', *, *, #1655, .T. ) ;
#4665=ORIENTED_EDGE ( 'NONE', *, *, #1477, .F. ) ;
#4666=CARTESIAN_POINT ( 'NONE',  ( 8.430890348300586368, 0.000000000000000000, -11.48836750521726913 ) ) ;
#4668=B_SPLINE_CURVE_WITH_KNOTS ( 'NONE', 3,
 ( #1112, #5306, #8475, #4081 ),
 .UNSPECIFIED., .F., .F.,
 ( 4, 4 ),
 ( 0.000000000000000000, 0.8452273900860258760 ),
 .UNSPECIFIED. ) ;
#4672=AXIS2_PLACEMENT_3D ( 'NONE', #5521, #5595, #8750 ) ;
#4675=EDGE_CURVE ( 'NONE', #205, #2665, #11893, .T. ) ;
#4677=CARTESIAN_POINT ( 'NONE',  ( 31.00000000000000000, 0.000000000000000000, 1.499999998612421725 ) ) ;
#4683=CARTESIAN_POINT ( 'NONE',  ( -5.733772933379541747, 0.000000000000000000, -13.04554897075796482 ) ) ;
#4688=ORIENTED_EDGE ( 'NONE', *, *, #4160, .F. ) ;
#4689=ORIENTED_EDGE ( 'NONE', *, *, #12348, .T. ) ;
#4694=CARTESIAN_POINT ( 'NONE',  ( 1.557181465540672161, 3.000000000000000000, -14.16466328168010591 ) ) ;
#4698=ORIENTED_EDGE ( 'NONE', *, *, #6502, .F. ) ;
#4704=B_SPLINE_CURVE_WITH_KNOTS ( 'NONE', 3,
 ( #6529, #4455, #11769, #7491 ),
 .UNSPECIFIED., .F., .F.,
 ( 4, 4 ),
 ( 0.000000000000000000, 0.8452273900860258760 ),
 .UNSPECIFIED. ) ;
#4705=ORIENTED_EDGE ( 'NONE', *, *, #11547, .T. ) ;
#4706=EDGE_CURVE ( 'NONE', #7580, #12590, #5752, .T. ) ;
#4708=CARTESIAN_POINT ( 'NONE',  ( -5.784789447945489549, 0.000000000000000000, 12.25836857253663581 ) ) ;
#4716=DIRECTION ( 'NONE',  ( -0.000000000000000000, -1.000000000000000000, -0.000000000000000000 ) ) ;
#4719=DIRECTION ( 'NONE',  ( 0.000000000000000000, 0.000000000000000000, 1.000000000000000000 ) ) ;
#4720=ORIENTED_EDGE ( 'NONE', *, *, #7101, .T. ) ;
#4728=DIRECTION ( 'NONE',  ( 0.000000000000000000, 0.000000000000000000, -1.000000000000000000 ) ) ;
#4732=LINE ( 'NONE', #2590, #10587 ) ;
#4740=EDGE_LOOP ( 'NONE', ( #7848, #2884, #7222, #3655 ) ) ;
#4754=ORIENTED_EDGE ( 'NONE', *, *, #8643, .F. ) ;
#4759=ORIENTED_EDGE ( 'NONE', *, *, #7932, .F. ) ;
#4760=CARTESIAN_POINT ( 'NONE',  ( -8.430890348300559722, 3.000000000000000000, 11.48836750521728689 ) ) ;
#4761=EDGE_CURVE ( 'NONE', #6683, #7859, #8731, .T. ) ;
#4763=B_SPLINE_CURVE_WITH_KNOTS ( 'NONE', 3,
 ( #7998, #11105, #6823, #7854 ),
 .UNSPECIFIED., .F., .F.,
 ( 4, 4 ),
 ( 0.1547128134717859205, 1.000000000000000000 ),
 .UNSPECIFIED. ) ;
#4764=ORIENTED_EDGE ( 'NONE', *, *, #7541, .T. ) ;
#4770=CARTESIAN_POINT ( 'NONE',  ( 2.568302020731520141, 3.000000000000000000, 12.56087513340552420 ) ) ;
#4772=EDGE_LOOP ( 'NONE', ( #4599, #13109, #12858, #8092 ) ) ;
#4775=EDGE_LOOP ( 'NONE', ( #251, #7512, #4156, #10074 ) ) ;
#4776=EDGE_CURVE ( 'NONE', #1924, #116, #11473, .T. ) ;
#4781=CARTESIAN_POINT ( 'NONE',  ( -13.04554897075796127, 3.000000000000000000, 5.733772933379547077 ) ) ;
#4790=ORIENTED_EDGE ( 'NONE', *, *, #2600, .T. ) ;
#4792=CARTESIAN_POINT ( 'NONE',  ( 13.04554897075798081, 0.000000000000000000, -5.733772933379503556 ) ) ;
#4794=LINE ( 'NONE', #8980, #13490 ) ;
#4795=CARTESIAN_POINT ( 'NONE',  ( 0.000000000000000000, 0.000000000000000000, 0.000000000000000000 ) ) ;
#4797=CARTESIAN_POINT ( 'NONE',  ( 31.00000000000000000, 3.000000000000000000, -1.500000000759764029 ) ) ;
#4802=ORIENTED_EDGE ( 'NONE', *, *, #9313, .F. ) ;
#4804=DIRECTION ( 'NONE',  ( 0.000000000000000000, 1.000000000000000000, 0.000000000000000000 ) ) ;
#4814=ORIENTED_EDGE ( 'NONE', *, *, #11409, .T. ) ;
#4818=ORIENTED_EDGE ( 'NONE', *, *, #5906, .T. ) ;
#4822=FACE_OUTER_BOUND ( 'NONE', #8349, .T. ) ;
#4826=CARTESIAN_POINT ( 'NONE',  ( 0.7901945867173618687, 0.000000000000000000, 12.78643498603817541 ) ) ;
#4827=CARTESIAN_POINT ( 'NONE',  ( -12.07793442604883971, 0.000000000000000000, 0.5400000000008015055 ) ) ;
#4838=AXIS2_PLACEMENT_3D ( 'NONE', #921, #9323, #2090 ) ;
#4842=CARTESIAN_POINT ( 'NONE',  ( 0.000000000000000000, 3.000000000000000000, 0.000000000000000000 ) ) ;
#4848=CARTESIAN_POINT ( 'NONE',  ( 11.13895890373327724, 0.000000000000000000, -7.723663868796764476 ) ) ;
#4849=CARTESIAN_POINT ( 'NONE',  ( -4.072642252455976219, 0.000000000000000000, -12.14623037080101398 ) ) ;
#4856=CIRCLE ( 'NONE', #10359, 1.499999999686092877 ) ;
#4857=CIRCLE ( 'NONE', #6832, 12.08999999999737440 ) ;
#4858=DIRECTION ( 'NONE',  ( 0.000000000000000000, 0.000000000000000000, 1.000000000000000000 ) ) ;
#4863=CARTESIAN_POINT ( 'NONE',  ( 8.504652361247167391, 0.000000000000000000, 9.593885948927674434 ) ) ;
#4866=VERTEX_POINT ( 'NONE', #12255 ) ;
#4868=CARTESIAN_POINT ( 'NONE',  ( -2.161962830978702677, 0.000000000000000000, 14.08504230442587435 ) ) ;
#4871=DIRECTION ( 'NONE',  ( 0.000000000000000000, 0.000000000000000000, -1.000000000000000000 ) ) ;
#4875=CARTESIAN_POINT ( 'NONE',  ( -11.48836750521723893, 3.000000000000000000, 8.430890348300625448 ) ) ;
#4876=DIRECTION ( 'NONE',  ( 0.000000000000000000, -0.000000000000000000, 1.000000000000000000 ) ) ;
#4877=CARTESIAN_POINT ( 'NONE',  ( -8.914835885878282795, 3.000000000000000000, -11.11702303352191556 ) ) ;
#4884=CARTESIAN_POINT ( 'NONE',  ( 6.506507307819716424, 0.000000000000000000, -10.18987059060247269 ) ) ;
#4889=EDGE_CURVE ( 'NONE', #2066, #688, #8351, .T. ) ;
#4891=EDGE_CURVE ( 'NONE', #846, #11264, #9914, .T. ) ;
#4892=DIRECTION ( 'NONE',  ( -0.000000000000000000, -1.000000000000000000, -0.000000000000000000 ) ) ;
#4896=ADVANCED_FACE ( 'NONE', ( #7005 ), #11348, .T. ) ;
#4901=CARTESIAN_POINT ( 'NONE',  ( 2.604531154829233586, 3.000000000000000000, 11.80612203322752585 ) ) ;
#4905=B_SPLINE_CURVE_WITH_KNOTS ( 'NONE', 3,
 ( #4012, #10286, #10222, #5943 ),
 .UNSPECIFIED., .F., .F.,
 ( 4, 4 ),
 ( 0.1547128134717859205, 1.000000000000000000 ),
 .UNSPECIFIED. ) ;
#4908=CARTESIAN_POINT ( 'NONE',  ( -1.557181465540221188, 3.000000000000000000, 14.16466328168015743 ) ) ;
#4913=CARTESIAN_POINT ( 'NONE',  ( 8.158651161643900807, 0.000000000000000000, 8.922136023539609440 ) ) ;
#4917=DIRECTION ( 'NONE',  ( 0.000000000000000000, 1.000000000000000000, 0.000000000000000000 ) ) ;
#4920=CARTESIAN_POINT ( 'NONE',  ( -10.18979803820068675, 3.000000000000000000, 6.506620931068438196 ) ) ;
#4923=FACE_OUTER_BOUND ( 'NONE', #7027, .T. ) ;
#4925=CIRCLE ( 'NONE', #2936, 1.500000000000000222 ) ;
#4938=B_SPLINE_CURVE_WITH_KNOTS ( 'NONE', 3,
 ( #5666, #9863, #12023, #10972 ),
 .UNSPECIFIED., .F., .F.,
 ( 4, 4 ),
 ( 0.2280192144657617603, 0.8452273900860258760 ),
 .UNSPECIFIED. ) ;
#4939=LINE ( 'NONE', #3010, #11756 ) ;
#4941=CARTESIAN_POINT ( 'NONE',  ( -0.7702044561450404059, 3.000000000000000000, 12.79759916868914793 ) ) ;
#4949=FACE_OUTER_BOUND ( 'NONE', #8473, .T. ) ;
#4950=VECTOR ( 'NONE', #30, 1000.000000000000000 ) ;
#4953=DIRECTION ( 'NONE',  ( 0.000000000000000000, 0.000000000000000000, 1.000000000000000000 ) ) ;
#4955=CARTESIAN_POINT ( 'NONE',  ( 5.797378255456016483, 0.000000000000000000, 12.25282671965375592 ) ) ;
#4960=ORIENTED_EDGE ( 'NONE', *, *, #6068, .T. ) ;
#4962=ORIENTED_EDGE ( 'NONE', *, *, #7501, .T. ) ;
#4963=VERTEX_POINT ( 'NONE', #4165 ) ;
#4973=CARTESIAN_POINT ( 'NONE',  ( -1.557181465540760534, 3.000000000000000000, -14.16466328168009703 ) ) ;
#4975=CARTESIAN_POINT ( 'NONE',  ( -2.604399508763951321, 3.000000000000000000, 11.80615107470197422 ) ) ;
#4977=EDGE_LOOP ( 'NONE', ( #5379, #5321, #11576, #10737 ) ) ;
#4982=ADVANCED_FACE ( 'NONE', ( #1139 ), #2157, .F. ) ;
#4983=CARTESIAN_POINT ( 'NONE',  ( 2.161962830978677363, 3.000000000000000000, 14.08504230442587613 ) ) ;
#4987=CARTESIAN_POINT ( 'NONE',  ( 0.000000000000000000, 0.000000000000000000, 0.000000000000000000 ) ) ;
#4992=DIRECTION ( 'NONE',  ( -9.145772869372436484E-17, 0.000000000000000000, -1.000000000000000000 ) ) ;
#4993=EDGE_CURVE ( 'NONE', #1111, #11851, #7265, .T. ) ;
#4996=VERTEX_POINT ( 'NONE', #1072 ) ;
#4997=EDGE_CURVE ( 'NONE', #655, #10050, #8562, .T. ) ;
#4999=ORIENTED_EDGE ( 'NONE', *, *, #12559, .F. ) ;
#5003=CARTESIAN_POINT ( 'NONE',  ( 0.000000000000000000, 3.000000000000000000, 0.000000000000000000 ) ) ;
#5006=CARTESIAN_POINT ( 'NONE',  ( -12.79759916868914615, 0.000000000000000000, -0.7702044561450367421 ) ) ;
#5007=EDGE_CURVE ( 'NONE', #9584, #9307, #5788, .T. ) ;
#5011=CARTESIAN_POINT ( 'NONE',  ( 10.72979803820132005, 0.000000000000000000, 5.571313494980133285 ) ) ;
#5015=CARTESIAN_POINT ( 'NONE',  ( -11.80615107470197778, 0.000000000000000000, -2.604399508763947768 ) ) ;
#5016=DIRECTION ( 'NONE',  ( -0.000000000000000000, -1.000000000000000000, -0.000000000000000000 ) ) ;
#5023=CARTESIAN_POINT ( 'NONE',  ( 2.414978278956333213, 0.000000000000000000, -13.33788847341978645 ) ) ;
#5025=ORIENTED_EDGE ( 'NONE', *, *, #10865, .T. ) ;
#5026=LINE ( 'NONE', #12206, #13029 ) ;
#5033=CARTESIAN_POINT ( 'NONE',  ( 0.000000000000000000, 0.000000000000000000, 0.000000000000000000 ) ) ;
#5034=DIRECTION ( 'NONE',  ( -0.000000000000000000, -1.000000000000000000, -0.000000000000000000 ) ) ;
#5045=CIRCLE ( 'NONE', #4602, 12.08999999999737440 ) ;
#5047=CARTESIAN_POINT ( 'NONE',  ( -5.733772933379472470, 0.000000000000000000, 13.04554897075799502 ) ) ;
#5053=DIRECTION ( 'NONE',  ( 0.000000000000000000, 0.000000000000000000, -1.000000000000000000 ) ) ;
#5065=AXIS2_PLACEMENT_3D ( 'NONE', #8217, #10354, #1302 ) ;
#5068=AXIS2_PLACEMENT_3D ( 'NONE', #9501, #4269, #4400 ) ;
#5070=EDGE_CURVE ( 'NONE', #525, #10812, #6639, .T. ) ;
#5074=B_SPLINE_CURVE_WITH_KNOTS ( 'NONE', 3,
 ( #1820, #5878, #11252, #9112 ),
 .UNSPECIFIED., .F., .F.,
 ( 4, 4 ),
 ( 0.1547128134717859205, 1.000000000000000000 ),
 .UNSPECIFIED. ) ;
#5079=ORIENTED_EDGE ( 'NONE', *, *, #4891, .F. ) ;
#5083=CARTESIAN_POINT ( 'NONE',  ( 1.557181465540669496, 3.000000000000000000, -14.16466328168010769 ) ) ;
#5089=CARTESIAN_POINT ( 'NONE',  ( 11.46847481510586775, 3.000000000000000000, 5.708888906988908829 ) ) ;
#5090=CARTESIAN_POINT ( 'NONE',  ( 2.546103534247748712, 0.000000000000000000, -12.55526518755974585 ) ) ;
#5100=DIRECTION ( 'NONE',  ( 0.000000000000000000, 1.000000000000000000, 0.000000000000000000 ) ) ;
#5101=CARTESIAN_POINT ( 'NONE',  ( -8.430890348300124515, 0.000000000000000000, 11.48836750521761019 ) ) ;
#5102=DIRECTION ( 'NONE',  ( 0.000000000000000000, 0.000000000000000000, 1.000000000000000000 ) ) ;
#5103=ORIENTED_EDGE ( 'NONE', *, *, #3200, .T. ) ;
#5105=DIRECTION ( 'NONE',  ( 0.000000000000000000, 1.000000000000000000, 0.000000000000000000 ) ) ;
#5106=AXIS2_PLACEMENT_3D ( 'NONE', #3405, #322, #12784 ) ;
#5110=B_SPLINE_CURVE_WITH_KNOTS ( 'NONE', 3,
 ( #6123, #4955, #825, #13497 ),
 .UNSPECIFIED., .F., .F.,
 ( 4, 4 ),
 ( 0.000000000000000000, 0.8452273900860258760 ),
 .UNSPECIFIED. ) ;
#5111=VERTEX_POINT ( 'NONE', #3532 ) ;
#5112=LINE ( 'NONE', #4983, #8895 ) ;
#5116=CARTESIAN_POINT ( 'NONE',  ( 8.430890348300625448, 3.000000000000000000, 11.48836750521723893 ) ) ;
#5118=CARTESIAN_POINT ( 'NONE',  ( -14.16466328168009881, 3.000000000000000000, 1.557181465540760534 ) ) ;
#5121=FACE_OUTER_BOUND ( 'NONE', #1179, .T. ) ;
#5127=EDGE_LOOP ( 'NONE', ( #4664, #5260, #9253, #9603 ) ) ;
#5132=VERTEX_POINT ( 'NONE', #5463 ) ;
#5134=CARTESIAN_POINT ( 'NONE',  ( -5.733772933379472470, 0.000000000000000000, 13.04554897075799502 ) ) ;
#5136=CYLINDRICAL_SURFACE ( 'NONE', #3162, 12.08999999999737263 ) ;
#5141=CARTESIAN_POINT ( 'NONE',  ( -10.67828022838850721, 3.000000000000000000, 7.077546079049267469 ) ) ;
#5144=CARTESIAN_POINT ( 'NONE',  ( -8.922136023539609440, 3.000000000000000000, 8.158651161643900807 ) ) ;
#5148=EDGE_CURVE ( 'NONE', #5785, #8320, #245, .T. ) ;
#5163=EDGE_CURVE ( 'NONE', #8924, #1247, #10775, .T. ) ;
#5180=ORIENTED_EDGE ( 'NONE', *, *, #11038, .T. ) ;
#5189=ORIENTED_EDGE ( 'NONE', *, *, #10821, .T. ) ;
#5195=DIRECTION ( 'NONE',  ( 0.000000000000000000, 0.000000000000000000, 1.000000000000000000 ) ) ;
#5197=CARTESIAN_POINT ( 'NONE',  ( -7.723663868796776910, 3.000000000000000000, -11.13895890373326303 ) ) ;
#5200=CARTESIAN_POINT ( 'NONE',  ( 8.922136023539611216, 3.000000000000000000, -8.158651161643899030 ) ) ;
#5205=EDGE_LOOP ( 'NONE', ( #5861, #13540, #1293, #12519 ) ) ;
#5206=ORIENTED_EDGE ( 'NONE', *, *, #11889, .F. ) ;
#5207=DIRECTION ( 'NONE',  ( -0.000000000000000000, -1.000000000000000000, -0.000000000000000000 ) ) ;
#5211=CARTESIAN_POINT ( 'NONE',  ( 8.430890348300565051, 3.000000000000000000, -11.48836750521728334 ) ) ;
#5213=DIRECTION ( 'NONE',  ( -0.000000000000000000, -1.000000000000000000, -0.000000000000000000 ) ) ;
#5216=DIRECTION ( 'NONE',  ( -0.000000000000000000, -1.000000000000000000, -0.000000000000000000 ) ) ;
#5222=EDGE_CURVE ( 'NONE', #1728, #6683, #7057, .T. ) ;
#5224=CARTESIAN_POINT ( 'NONE',  ( 12.90250726680438476, 0.000000000000000000, 4.728042766759046778 ) ) ;
#5234=FACE_OUTER_BOUND ( 'NONE', #3158, .T. ) ;
#5236=ADVANCED_FACE ( 'NONE', ( #1902 ), #6329, .F. ) ;
#5241=DIRECTION ( 'NONE',  ( 0.000000000000000000, 0.000000000000000000, 1.000000000000000000 ) ) ;
#5245=VERTEX_POINT ( 'NONE', #9182 ) ;
#5248=DIRECTION ( 'NONE',  ( -0.000000000000000000, -1.000000000000000000, -0.000000000000000000 ) ) ;
#5255=CARTESIAN_POINT ( 'NONE',  ( -7.077546079049271910, 0.000000000000000000, -10.67828022838850544 ) ) ;
#5260=ORIENTED_EDGE ( 'NONE', *, *, #7985, .F. ) ;
#5264=EDGE_CURVE ( 'NONE', #8754, #9963, #8570, .T. ) ;
#5266=CARTESIAN_POINT ( 'NONE',  ( 5.170206418547604876, 0.000000000000000000, -13.27898586450069196 ) ) ;
#5270=AXIS2_PLACEMENT_3D ( 'NONE', #11640, #10536, #11704 ) ;
#5278=CIRCLE ( 'NONE', #10992, 14.25000000000000178 ) ;
#5279=FACE_OUTER_BOUND ( 'NONE', #3556, .T. ) ;
#5283=CARTESIAN_POINT ( 'NONE',  ( 0.000000000000000000, 0.000000000000000000, 0.000000000000000000 ) ) ;
#5285=DIRECTION ( 'NONE',  ( 0.000000000000000000, 1.000000000000000000, 0.000000000000000000 ) ) ;
#5286=VECTOR ( 'NONE', #602, 1000.000000000000000 ) ;
#5287=ORIENTED_EDGE ( 'NONE', *, *, #6955, .T. ) ;
#5297=CARTESIAN_POINT ( 'NONE',  ( 5.784789447945496654, 0.000000000000000000, -12.25836857253663581 ) ) ;
#5299=LINE ( 'NONE', #10804, #3828 ) ;
#5302=ORIENTED_EDGE ( 'NONE', *, *, #6725, .F. ) ;
#5304=ORIENTED_EDGE ( 'NONE', *, *, #8912, .T. ) ;
#5306=CARTESIAN_POINT ( 'NONE',  ( -8.771102293099080072, 0.000000000000000000, -10.33484986938307770 ) ) ;
#5311=CYLINDRICAL_SURFACE ( 'NONE', #12873, 12.08999999999737440 ) ;
#5321=ORIENTED_EDGE ( 'NONE', *, *, #13340, .F. ) ;
#5322=CARTESIAN_POINT ( 'NONE',  ( 13.04554897075796838, 3.000000000000000000, -5.733772933379540859 ) ) ;
#5330=CIRCLE ( 'NONE', #12821, 14.25000000000000178 ) ;
#5333=EDGE_CURVE ( 'NONE', #5245, #3720, #11880, .T. ) ;
#5338=VECTOR ( 'NONE', #611, 1000.000000000000000 ) ;
#5353=CARTESIAN_POINT ( 'NONE',  ( 12.90250726680438476, 0.000000000000000000, 4.728042766759046778 ) ) ;
#5365=CIRCLE ( 'NONE', #8438, 1.499999999686092877 ) ;
#5367=CARTESIAN_POINT ( 'NONE',  ( 5.170206418547604876, 3.000000000000000000, -13.27898586450069196 ) ) ;
#5369=DIRECTION ( 'NONE',  ( 0.000000000000000000, 0.000000000000000000, -1.000000000000000000 ) ) ;
#5371=CARTESIAN_POINT ( 'NONE',  ( -5.170206418547117266, 3.000000000000000000, 13.27898586450088203 ) ) ;
#5373=EDGE_CURVE ( 'NONE', #846, #1437, #4020, .T. ) ;
#5379=ORIENTED_EDGE ( 'NONE', *, *, #2613, .T. ) ;
#5391=DIRECTION ( 'NONE',  ( 1.370446048119726253E-16, -0.000000000000000000, 1.000000000000000000 ) ) ;
#5392=ADVANCED_FACE ( 'NONE', ( #7202 ), #11643, .T. ) ;
#5404=CARTESIAN_POINT ( 'NONE',  ( 8.914835885878215294, 3.000000000000000000, 11.11702303352197418 ) ) ;
#5405=CARTESIAN_POINT ( 'NONE',  ( -10.67828022838850721, 0.000000000000000000, 7.077546079049267469 ) ) ;
#5407=DIRECTION ( 'NONE',  ( 0.000000000000000000, 0.000000000000000000, -1.000000000000000000 ) ) ;
#5410=ORIENTED_EDGE ( 'NONE', *, *, #3659, .T. ) ;
#5413=B_SPLINE_CURVE_WITH_KNOTS ( 'NONE', 3,
 ( #7723, #4495, #12906, #3450 ),
 .UNSPECIFIED., .F., .F.,
 ( 4, 4 ),
 ( 0.000000000000000000, 0.8452273900860258760 ),
 .UNSPECIFIED. ) ;
#5417=CARTESIAN_POINT ( 'NONE',  ( 0.000000000000000000, 3.000000000000000000, 0.000000000000000000 ) ) ;
#5418=CARTESIAN_POINT ( 'NONE',  ( 5.571313494980132397, 3.000000000000000000, -10.72979803820131472 ) ) ;
#5419=B_SPLINE_CURVE_WITH_KNOTS ( 'NONE', 3,
 ( #3077, #3215, #6180, #10460 ),
 .UNSPECIFIED., .F., .F.,
 ( 4, 4 ),
 ( 0.1547128134717859205, 1.000000000000000000 ),
 .UNSPECIFIED. ) ;
#5420=DIRECTION ( 'NONE',  ( -0.000000000000000000, -1.000000000000000000, -0.000000000000000000 ) ) ;
#5422=FACE_OUTER_BOUND ( 'NONE', #4481, .T. ) ;
#5423=EDGE_LOOP ( 'NONE', ( #566, #11759, #5968, #10470 ) ) ;
#5431=DIRECTION ( 'NONE',  ( 0.000000000000000000, 1.000000000000000000, 0.000000000000000000 ) ) ;
#5441=VERTEX_POINT ( 'NONE', #11949 ) ;
#5444=AXIS2_PLACEMENT_3D ( 'NONE', #6621, #8743, #12958 ) ;
#5449=DIRECTION ( 'NONE',  ( 0.000000000000000000, 1.000000000000000000, 0.000000000000000000 ) ) ;
#5450=DIRECTION ( 'NONE',  ( -0.000000000000000000, -1.000000000000000000, -0.000000000000000000 ) ) ;
#5453=ORIENTED_EDGE ( 'NONE', *, *, #4130, .F. ) ;
#5454=DIRECTION ( 'NONE',  ( 0.000000000000000000, 0.000000000000000000, 1.000000000000000000 ) ) ;
#5463=CARTESIAN_POINT ( 'NONE',  ( 31.00000000000000000, 3.000000000000000000, -4.000000001073670930 ) ) ;
#5470=ADVANCED_FACE ( 'NONE', ( #10012 ), #6710, .T. ) ;
#5472=ORIENTED_EDGE ( 'NONE', *, *, #987, .F. ) ;
#5479=AXIS2_PLACEMENT_3D ( 'NONE', #7423, #2180, #11421 ) ;
#5480=CARTESIAN_POINT ( 'NONE',  ( 0.000000000000000000, 0.000000000000000000, 0.000000000000000000 ) ) ;
#5493=EDGE_CURVE ( 'NONE', #2347, #13326, #5713, .T. ) ;
#5502=VERTEX_POINT ( 'NONE', #1753 ) ;
#5503=ORIENTED_EDGE ( 'NONE', *, *, #12770, .T. ) ;
#5505=DIRECTION ( 'NONE',  ( 0.000000000000000000, 0.000000000000000000, 1.000000000000000000 ) ) ;
#5510=VECTOR ( 'NONE', #2654, 1000.000000000000000 ) ;
#5511=LINE ( 'NONE', #4283, #1424 ) ;
#5517=CARTESIAN_POINT ( 'NONE',  ( -11.46814821560793440, 0.000000000000000000, 5.731782959214994477 ) ) ;
#5520=AXIS2_PLACEMENT_3D ( 'NONE', #3398, #11672, #7609 ) ;
#5521=CARTESIAN_POINT ( 'NONE',  ( 0.000000000000000000, 0.000000000000000000, 0.000000000000000000 ) ) ;
#5523=AXIS2_PLACEMENT_3D ( 'NONE', #5003, #3961, #12391 ) ;
#5529=VECTOR ( 'NONE', #6697, 1000.000000000000000 ) ;
#5533=CARTESIAN_POINT ( 'NONE',  ( 8.430890348300625448, 0.000000000000000000, 11.48836750521723893 ) ) ;
#5541=B_SPLINE_SURFACE_WITH_KNOTS ( 'NONE', 3, 1, ( 
 ( #12107, #2456 ),
 ( #6727, #8921 ),
 ( #9958, #10928 ),
 ( #6938, #11970 ) ),
 .UNSPECIFIED., .F., .F., .F.,
 ( 4, 4 ),
 ( 2, 2 ),
 ( 0.1547128134717859205, 0.7774895956119340923 ),
 ( 0.000000000000000000, 1.000000000000000000 ),
 .UNSPECIFIED. ) ;
#5547=CARTESIAN_POINT ( 'NONE',  ( -12.07794044664754018, 3.000000000000000000, -0.5398653231797256868 ) ) ;
#5549=CIRCLE ( 'NONE', #4672, 14.25000000000000178 ) ;
#5551=CARTESIAN_POINT ( 'NONE',  ( -11.46814821560793440, 3.000000000000000000, 5.731782959214994477 ) ) ;
#5553=CARTESIAN_POINT ( 'NONE',  ( -10.72973591378220348, 0.000000000000000000, 5.571433138827830867 ) ) ;
#5555=EDGE_CURVE ( 'NONE', #1728, #13138, #11553, .T. ) ;
#5558=ORIENTED_EDGE ( 'NONE', *, *, #4646, .F. ) ;
#5562=EDGE_CURVE ( 'NONE', #1090, #12859, #8359, .T. ) ;
#5563=ORIENTED_EDGE ( 'NONE', *, *, #5581, .T. ) ;
#5567=CARTESIAN_POINT ( 'NONE',  ( -10.18979803820068675, 3.000000000000000000, 6.506620931068438196 ) ) ;
#5572=CARTESIAN_POINT ( 'NONE',  ( -11.80612203322752585, 0.000000000000000000, 2.604531154829235362 ) ) ;
#5574=ORIENTED_EDGE ( 'NONE', *, *, #6917, .T. ) ;
#5577=ORIENTED_EDGE ( 'NONE', *, *, #2731, .F. ) ;
#5578=UNCERTAINTY_MEASURE_WITH_UNIT (LENGTH_MEASURE( 1.000000000000000082E-05 ), #4339, 'distance_accuracy_value', 'NONE');
#5581=EDGE_CURVE ( 'NONE', #4662, #5132, #12342, .T. ) ;
#5586=CARTESIAN_POINT ( 'NONE',  ( 2.546103534247748712, 3.000000000000000000, -12.55526518755974585 ) ) ;
#5587=DIRECTION ( 'NONE',  ( 0.000000000000000000, 1.000000000000000000, 0.000000000000000000 ) ) ;
#5589=ADVANCED_FACE ( 'NONE', ( #4089 ), #3329, .F. ) ;
#5595=DIRECTION ( 'NONE',  ( 0.000000000000000000, 1.000000000000000000, 0.000000000000000000 ) ) ;
#5600=ORIENTED_EDGE ( 'NONE', *, *, #4891, .T. ) ;
#5604=CARTESIAN_POINT ( 'NONE',  ( 3.647470871583629926, 3.000000000000000000, -11.52666717836884125 ) ) ;
#5607=EDGE_CURVE ( 'NONE', #1734, #2852, #5940, .T. ) ;
#5610=EDGE_CURVE ( 'NONE', #10338, #688, #7259, .T. ) ;
#5618=LINE ( 'NONE', #11826, #2062 ) ;
#5620=EDGE_CURVE ( 'NONE', #10439, #597, #1767, .T. ) ;
#5622=CARTESIAN_POINT ( 'NONE',  ( -12.07793442604884682, 0.000000000000000000, 0.5400000000005513723 ) ) ;
#5628=EDGE_LOOP ( 'NONE', ( #13163, #8419, #5710, #575 ) ) ;
#5629=ORIENTED_EDGE ( 'NONE', *, *, #2484, .F. ) ;
#5638=CARTESIAN_POINT ( 'NONE',  ( 5.733772933379474246, 3.000000000000000000, -13.04554897075799502 ) ) ;
#5639=CARTESIAN_POINT ( 'NONE',  ( 8.482622935103764306, 3.000000000000000000, -9.600126836553261711 ) ) ;
#5647=ORIENTED_EDGE ( 'NONE', *, *, #1207, .F. ) ;
#5648=EDGE_CURVE ( 'NONE', #3799, #6616, #6148, .T. ) ;
#5649=ORIENTED_EDGE ( 'NONE', *, *, #7105, .F. ) ;
#5658=CARTESIAN_POINT ( 'NONE',  ( 31.00000000000000000, 0.000000000000000000, -4.000000001073670930 ) ) ;
#5664=EDGE_LOOP ( 'NONE', ( #7033, #2609, #3630, #4185 ) ) ;
#5666=CARTESIAN_POINT ( 'NONE',  ( 13.27898586450067420, 3.000000000000000000, 5.170206418547648397 ) ) ;
#5671=DIRECTION ( 'NONE',  ( 0.000000000000000000, 1.000000000000000000, 0.000000000000000000 ) ) ;
#5675=VERTEX_POINT ( 'NONE', #4677 ) ;
#5676=ADVANCED_FACE ( 'NONE', ( #11731, #12703, #1508 ), #8863, .T. ) ;
#5679=LINE ( 'NONE', #7879, #12843 ) ;
#5684=CARTESIAN_POINT ( 'NONE',  ( 0.000000000000000000, 3.000000000000000000, 0.000000000000000000 ) ) ;
#5686=DIRECTION ( 'NONE',  ( 0.000000000000000000, 0.000000000000000000, -1.000000000000000000 ) ) ;
#5687=CARTESIAN_POINT ( 'NONE',  ( 8.914835885878220623, 0.000000000000000000, -11.11702303352196708 ) ) ;
#5691=ORIENTED_EDGE ( 'NONE', *, *, #8708, .T. ) ;
#5693=B_SPLINE_CURVE_WITH_KNOTS ( 'NONE', 3,
 ( #7464, #7530, #10904, #11738 ),
 .UNSPECIFIED., .F., .F.,
 ( 4, 4 ),
 ( 0.1547128134717859205, 1.000000000000000000 ),
 .UNSPECIFIED. ) ;
#5696=CARTESIAN_POINT ( 'NONE',  ( 11.14709020439929787, 3.000000000000000000, 7.712570079660892475 ) ) ;
#5698=CARTESIAN_POINT ( 'NONE',  ( -2.604399508763953985, 3.000000000000000000, 11.80615107470197778 ) ) ;
#5701=CYLINDRICAL_SURFACE ( 'NONE', #12229, 12.08999999999737440 ) ;
#5702=ORIENTED_EDGE ( 'NONE', *, *, #1991, .T. ) ;
#5706=PRODUCT_DEFINITION ( 'UNKNOWN', '', #13112, #11920 ) ;
#5710=ORIENTED_EDGE ( 'NONE', *, *, #6023, .F. ) ;
#5712=DIRECTION ( 'NONE',  ( 1.000000000000000000, 0.000000000000000000, 0.000000000000000000 ) ) ;
#5713=CIRCLE ( 'NONE', #6605, 14.25000000000000355 ) ;
#5718=FACE_OUTER_BOUND ( 'NONE', #7463, .T. ) ;
#5721=EDGE_CURVE ( 'NONE', #3089, #9203, #8150, .T. ) ;
#5723=EDGE_CURVE ( 'NONE', #3444, #13127, #6800, .T. ) ;
#5728=ORIENTED_EDGE ( 'NONE', *, *, #2731, .T. ) ;
#5733=CARTESIAN_POINT ( 'NONE',  ( 3.647470871583629926, 0.000000000000000000, -11.52666717836884125 ) ) ;
#5734=CARTESIAN_POINT ( 'NONE',  ( -14.08504230442586369, 0.000000000000000000, 2.161962830978784389 ) ) ;
#5737=CARTESIAN_POINT ( 'NONE',  ( 6.506507307819716424, 0.000000000000000000, -10.18987059060247269 ) ) ;
#5738=VECTOR ( 'NONE', #7673, 1000.000000000000000 ) ;
#5742=ADVANCED_FACE ( 'NONE', ( #7396 ), #10053, .F. ) ;
#5747=EDGE_CURVE ( 'NONE', #3799, #2502, #2006, .T. ) ;
#5749=CARTESIAN_POINT ( 'NONE',  ( 5.733772933379541747, 0.000000000000000000, 13.04554897075796482 ) ) ;
#5752=LINE ( 'NONE', #12931, #3306 ) ;
#5756=ADVANCED_FACE ( 'NONE', ( #8482 ), #7959, .F. ) ;
#5760=ORIENTED_EDGE ( 'NONE', *, *, #3722, .F. ) ;
#5763=FACE_OUTER_BOUND ( 'NONE', #9983, .T. ) ;
#5768=VECTOR ( 'NONE', #3947, 1000.000000000000000 ) ;
#5769=CARTESIAN_POINT ( 'NONE',  ( -11.11702303352192445, 3.000000000000000000, 8.914835885878272137 ) ) ;
#5775=FACE_OUTER_BOUND ( 'NONE', #3138, .T. ) ;
#5778=AXIS2_PLACEMENT_3D ( 'NONE', #3558, #4461, #1236 ) ;
#5783=CARTESIAN_POINT ( 'NONE',  ( 7.712570079660896916, 0.000000000000000000, -11.14709020439929432 ) ) ;
#5785=VERTEX_POINT ( 'NONE', #12410 ) ;
#5788=B_SPLINE_CURVE_WITH_KNOTS ( 'NONE', 3,
 ( #185, #8559, #2042, #11476 ),
 .UNSPECIFIED., .F., .F.,
 ( 4, 4 ),
 ( 0.000000000000000000, 0.8452273900860258760 ),
 .UNSPECIFIED. ) ;
#5789=VECTOR ( 'NONE', #1333, 1000.000000000000000 ) ;
#5792=FACE_OUTER_BOUND ( 'NONE', #5628, .T. ) ;
#5794=DIRECTION ( 'NONE',  ( 0.000000000000000000, 1.000000000000000000, 0.000000000000000000 ) ) ;
#5799=ORIENTED_EDGE ( 'NONE', *, *, #8171, .T. ) ;
#5805=DIRECTION ( 'NONE',  ( 0.000000000000000000, 0.000000000000000000, 1.000000000000000000 ) ) ;
#5817=DIRECTION ( 'NONE',  ( -0.000000000000000000, -1.000000000000000000, -0.000000000000000000 ) ) ;
#5818=CARTESIAN_POINT ( 'NONE',  ( -1.557181465540760534, 0.000000000000000000, -14.16466328168009703 ) ) ;
#5825=ORIENTED_EDGE ( 'NONE', *, *, #9550, .F. ) ;
#5830=CARTESIAN_POINT ( 'NONE',  ( -14.08504230442586369, 3.000000000000000000, 2.161962830978781724 ) ) ;
#5834=AXIS2_PLACEMENT_3D ( 'NONE', #11781, #12948, #1178 ) ;
#5835=EDGE_CURVE ( 'NONE', #4996, #10780, #10182, .T. ) ;
#5836=DIRECTION ( 'NONE',  ( 0.000000000000000000, 0.000000000000000000, 1.000000000000000000 ) ) ;
#5841=DIRECTION ( 'NONE',  ( 0.000000000000000000, 0.000000000000000000, 1.000000000000000000 ) ) ;
#5842=ORIENTED_EDGE ( 'NONE', *, *, #1526, .T. ) ;
#5843=( GEOMETRIC_REPRESENTATION_CONTEXT ( 3 ) GLOBAL_UNCERTAINTY_ASSIGNED_CONTEXT ( ( #12063 ) ) GLOBAL_UNIT_ASSIGNED_CONTEXT ( ( #8067, #11505, #13512 ) ) REPRESENTATION_CONTEXT ( 'NONE', 'WORKASPACE' ) );
#5844=CARTESIAN_POINT ( 'NONE',  ( -2.604531154829235362, 0.000000000000000000, -11.80612203322752585 ) ) ;
#5851=B_SPLINE_CURVE_WITH_KNOTS ( 'NONE', 3,
 ( #13137, #12935, #8986, #2459 ),
 .UNSPECIFIED., .F., .F.,
 ( 4, 4 ),
 ( 0.1547128134717859205, 0.7774895956119340923 ),
 .UNSPECIFIED. ) ;
#5859=CARTESIAN_POINT ( 'NONE',  ( 8.760376775873721655, 0.000000000000000000, -10.34346111134700585 ) ) ;
#5861=ORIENTED_EDGE ( 'NONE', *, *, #11561, .T. ) ;
#5862=EDGE_CURVE ( 'NONE', #12859, #1887, #2984, .T. ) ;
#5867=CARTESIAN_POINT ( 'NONE',  ( -12.78643498603817896, 3.000000000000000000, 0.7901945867173603144 ) ) ;
#5869=DIRECTION ( 'NONE',  ( 0.000000000000000000, 0.000000000000000000, 1.000000000000000000 ) ) ;
#5872=ORIENTED_EDGE ( 'NONE', *, *, #4482, .F. ) ;
#5873=ORIENTED_EDGE ( 'NONE', *, *, #6422, .F. ) ;
#5878=CARTESIAN_POINT ( 'NONE',  ( -12.55526518755974585, 3.000000000000000000, -2.546103534247746047 ) ) ;
#5879=CARTESIAN_POINT ( 'NONE',  ( -8.158651161643904359, 0.000000000000000000, -8.922136023539605887 ) ) ;
#5885=CARTESIAN_POINT ( 'NONE',  ( -2.161962830978783057, 0.000000000000000000, -14.08504230442586369 ) ) ;
#5888=ORIENTED_EDGE ( 'NONE', *, *, #3282, .F. ) ;
#5889=EDGE_CURVE ( 'NONE', #6233, #12697, #9902, .T. ) ;
#5893=CARTESIAN_POINT ( 'NONE',  ( 31.00000000000000000, 0.000000000000000000, -1.073670993220974656E-09 ) ) ;
#5894=DIRECTION ( 'NONE',  ( -0.000000000000000000, -1.000000000000000000, -0.000000000000000000 ) ) ;
#5900=VERTEX_POINT ( 'NONE', #4875 ) ;
#5903=LINE ( 'NONE', #545, #6227 ) ;
#5906=EDGE_CURVE ( 'NONE', #5900, #9964, #9420, .T. ) ;
#5907=CYLINDRICAL_SURFACE ( 'NONE', #11870, 12.08999999999737440 ) ;
#5911=DIRECTION ( 'NONE',  ( 0.000000000000000000, 0.000000000000000000, 1.000000000000000000 ) ) ;
#5913=DIRECTION ( 'NONE',  ( 0.000000000000000000, 0.000000000000000000, -1.000000000000000000 ) ) ;
#5916=EDGE_CURVE ( 'NONE', #9457, #8093, #6380, .T. ) ;
#5917=VERTEX_POINT ( 'NONE', #12602 ) ;
#5921=CARTESIAN_POINT ( 'NONE',  ( -13.04554897075795949, 3.000000000000000000, 5.733772933379550629 ) ) ;
#5929=FACE_OUTER_BOUND ( 'NONE', #10937, .T. ) ;
#5933=DIRECTION ( 'NONE',  ( 0.000000000000000000, 1.000000000000000000, 0.000000000000000000 ) ) ;
#5934=EDGE_CURVE ( 'NONE', #10050, #9874, #7252, .T. ) ;
#5936=ADVANCED_FACE ( 'NONE', ( #12730 ), #7628, .F. ) ;
#5940=CIRCLE ( 'NONE', #14, 12.08999999999737263 ) ;
#5941=CIRCLE ( 'NONE', #3284, 12.08999999999737440 ) ;
#5942=CARTESIAN_POINT ( 'NONE',  ( 8.771102293099069414, 3.000000000000000000, 10.33484986938308303 ) ) ;
#5943=CARTESIAN_POINT ( 'NONE',  ( 11.48836750521724070, 3.000000000000000000, -8.430890348300621895 ) ) ;
#5949=DIRECTION ( 'NONE',  ( -0.000000000000000000, -1.000000000000000000, -0.000000000000000000 ) ) ;
#5954=ORIENTED_EDGE ( 'NONE', *, *, #4997, .T. ) ;
#5959=DIRECTION ( 'NONE',  ( -0.000000000000000000, -1.000000000000000000, -0.000000000000000000 ) ) ;
#5961=VECTOR ( 'NONE', #139, 1000.000000000000000 ) ;
#5964=CARTESIAN_POINT ( 'NONE',  ( 0.000000000000000000, 3.000000000000000000, 0.000000000000000000 ) ) ;
#5968=ORIENTED_EDGE ( 'NONE', *, *, #8504, .F. ) ;
#5969=CIRCLE ( 'NONE', #9700, 14.25000000000000178 ) ;
#5973=ORIENTED_EDGE ( 'NONE', *, *, #1701, .T. ) ;
#5974=CARTESIAN_POINT ( 'NONE',  ( -2.161962830978785277, 3.000000000000000000, -14.08504230442586369 ) ) ;
#5981=ADVANCED_FACE ( 'NONE', ( #11626 ), #6633, .F. ) ;
#5987=DIRECTION ( 'NONE',  ( 0.000000000000000000, 0.000000000000000000, 1.000000000000000000 ) ) ;
#6003=DIRECTION ( 'NONE',  ( -0.000000000000000000, -1.000000000000000000, -0.000000000000000000 ) ) ;
#6007=DIRECTION ( 'NONE',  ( 0.000000000000000000, 1.000000000000000000, 0.000000000000000000 ) ) ;
#6008=ORIENTED_EDGE ( 'NONE', *, *, #4482, .T. ) ;
#6009=CARTESIAN_POINT ( 'NONE',  ( -5.733772933379472470, 3.000000000000000000, 13.04554897075799502 ) ) ;
#6010=EDGE_CURVE ( 'NONE', #3195, #8124, #11010, .T. ) ;
#6012=ORIENTED_EDGE ( 'NONE', *, *, #4556, .F. ) ;
#6016=AXIS2_PLACEMENT_3D ( 'NONE', #3813, #4917, #6025 ) ;
#6020=FACE_OUTER_BOUND ( 'NONE', #1909, .T. ) ;
#6021=EDGE_CURVE ( 'NONE', #525, #4274, #1170, .T. ) ;
#6022=CARTESIAN_POINT ( 'NONE',  ( -13.04554897075795949, 0.000000000000000000, 5.733772933379550629 ) ) ;
#6023=EDGE_CURVE ( 'NONE', #3853, #5675, #4856, .T. ) ;
#6025=DIRECTION ( 'NONE',  ( 0.000000000000000000, 0.000000000000000000, 1.000000000000000000 ) ) ;
#6027=CARTESIAN_POINT ( 'NONE',  ( 5.797378255456016483, 3.000000000000000000, 12.25282671965375592 ) ) ;
#6033=B_SPLINE_CURVE_WITH_KNOTS ( 'NONE', 3,
 ( #7690, #397, #669, #605 ),
 .UNSPECIFIED., .F., .F.,
 ( 4, 4 ),
 ( 0.000000000000000000, 0.8452273900860258760 ),
 .UNSPECIFIED. ) ;
#6034=ORIENTED_EDGE ( 'NONE', *, *, #2961, .F. ) ;
#6040=DIRECTION ( 'NONE',  ( 0.000000000000000000, 1.000000000000000000, 0.000000000000000000 ) ) ;
#6042=EDGE_CURVE ( 'NONE', #357, #12112, #2148, .T. ) ;
#6048=CIRCLE ( 'NONE', #8025, 14.25000000000000000 ) ;
#6051=ORIENTED_EDGE ( 'NONE', *, *, #11459, .F. ) ;
#6055=CARTESIAN_POINT ( 'NONE',  ( -2.568302020731516588, 0.000000000000000000, -12.56087513340552242 ) ) ;
#6058=DIRECTION ( 'NONE',  ( 0.000000000000000000, 1.000000000000000000, 0.000000000000000000 ) ) ;
#6059=CARTESIAN_POINT ( 'NONE',  ( 7.065816209474156118, 3.000000000000000000, -10.69794375946289833 ) ) ;
#6060=CARTESIAN_POINT ( 'NONE',  ( -11.11702303352191734, 3.000000000000000000, 8.914835885878279242 ) ) ;
#6066=ORIENTED_EDGE ( 'NONE', *, *, #11561, .F. ) ;
#6068=EDGE_CURVE ( 'NONE', #1235, #8499, #3457, .T. ) ;
#6073=CARTESIAN_POINT ( 'NONE',  ( 7.065816209474156118, 3.000000000000000000, -10.69794375946289833 ) ) ;
#6076=CARTESIAN_POINT ( 'NONE',  ( -11.80615107470192804, 3.000000000000000000, -2.604399508764160487 ) ) ;
#6084=EDGE_CURVE ( 'NONE', #7786, #597, #3547, .T. ) ;
#6093=CARTESIAN_POINT ( 'NONE',  ( -5.170206418547117266, 3.000000000000000000, 13.27898586450088203 ) ) ;
#6097=DIRECTION ( 'NONE',  ( -0.000000000000000000, -1.000000000000000000, -0.000000000000000000 ) ) ;
#6098=CARTESIAN_POINT ( 'NONE',  ( 10.72973591378220704, 0.000000000000000000, -5.571433138827823761 ) ) ;
#6101=EDGE_CURVE ( 'NONE', #8926, #8654, #394, .T. ) ;
#6102=ORIENTED_EDGE ( 'NONE', *, *, #8436, .F. ) ;
#6110=CARTESIAN_POINT ( 'NONE',  ( 12.25282671965375592, 3.000000000000000000, -5.797378255456012930 ) ) ;
#6112=B_SPLINE_SURFACE_WITH_KNOTS ( 'NONE', 3, 1, ( 
 ( #3166, #277 ),
 ( #11641, #4468 ),
 ( #4194, #5297 ),
 ( #7440, #2075 ) ),
 .UNSPECIFIED., .F., .F., .F.,
 ( 4, 4 ),
 ( 2, 2 ),
 ( 0.1547128134717859205, 1.000000000000000000 ),
 ( 0.000000000000000000, 1.000000000000000000 ),
 .UNSPECIFIED. ) ;
#6115=EDGE_CURVE ( 'NONE', #9457, #8335, #11462, .T. ) ;
#6117=ORIENTED_EDGE ( 'NONE', *, *, #7932, .T. ) ;
#6121=CARTESIAN_POINT ( 'NONE',  ( 0.5398653231797245766, 3.000000000000000000, -12.07794044664754018 ) ) ;
#6122=DIRECTION ( 'NONE',  ( -0.000000000000000000, -1.000000000000000000, -0.000000000000000000 ) ) ;
#6123=CARTESIAN_POINT ( 'NONE',  ( 5.733772933379453818, 0.000000000000000000, 13.04554897075800568 ) ) ;
#6132=CARTESIAN_POINT ( 'NONE',  ( 0.000000000000000000, 3.000000000000000000, 0.000000000000000000 ) ) ;
#6135=CARTESIAN_POINT ( 'NONE',  ( -14.08504230442586369, 3.000000000000000000, 2.161962830978781724 ) ) ;
#6136=EDGE_CURVE ( 'NONE', #1887, #7786, #684, .T. ) ;
#6139=ORIENTED_EDGE ( 'NONE', *, *, #7532, .F. ) ;
#6145=CARTESIAN_POINT ( 'NONE',  ( -11.80612203322752585, 3.000000000000000000, 2.604531154829235362 ) ) ;
#6146=DIRECTION ( 'NONE',  ( 0.000000000000000000, 1.000000000000000000, 0.000000000000000000 ) ) ;
#6147=AXIS2_PLACEMENT_3D ( 'NONE', #11689, #2120, #6378 ) ;
#6148=LINE ( 'NONE', #8215, #1995 ) ;
#6150=CARTESIAN_POINT ( 'NONE',  ( 31.00000000000000000, 0.000000000000000000, -1.073670993220974656E-09 ) ) ;
#6151=DIRECTION ( 'NONE',  ( -0.000000000000000000, -1.000000000000000000, -0.000000000000000000 ) ) ;
#6154=EDGE_CURVE ( 'NONE', #2645, #8456, #13499, .T. ) ;
#6155=ORIENTED_EDGE ( 'NONE', *, *, #8168, .T. ) ;
#6168=EDGE_CURVE ( 'NONE', #11807, #4282, #12039, .T. ) ;
#6169=DIRECTION ( 'NONE',  ( 0.000000000000000000, 0.000000000000000000, 1.000000000000000000 ) ) ;
#6176=CARTESIAN_POINT ( 'NONE',  ( 10.18979803820051622, 3.000000000000000000, -6.506620931068703761 ) ) ;
#6177=CARTESIAN_POINT ( 'NONE',  ( 0.000000000000000000, 3.000000000000000000, 0.000000000000000000 ) ) ;
#6180=CARTESIAN_POINT ( 'NONE',  ( -4.577511697546077230, 3.000000000000000000, -12.75843939030334795 ) ) ;
#6184=EDGE_CURVE ( 'NONE', #3598, #7142, #6786, .T. ) ;
#6191=ORIENTED_EDGE ( 'NONE', *, *, #3314, .T. ) ;
#6197=FILL_AREA_STYLE ('',( #4191 ) ) ;
#6199=CARTESIAN_POINT ( 'NONE',  ( -3.647599401157625376, 3.000000000000000000, -11.52662650599085836 ) ) ;
#6200=EDGE_CURVE ( 'NONE', #6731, #523, #12018, .T. ) ;
#6203=LINE ( 'NONE', #6135, #12661 ) ;
#6208=EDGE_LOOP ( 'NONE', ( #733, #9645, #2584, #10646 ) ) ;
#6210=CARTESIAN_POINT ( 'NONE',  ( 1.836970198721030181E-16, 3.000000000000000000, 1.500000000000000222 ) ) ;
#6211=ORIENTED_EDGE ( 'NONE', *, *, #1477, .T. ) ;
#6212=EDGE_CURVE ( 'NONE', #9781, #5917, #6936, .T. ) ;
#6214=AXIS2_PLACEMENT_3D ( 'NONE', #6688, #1312, #5505 ) ;
#6218=CARTESIAN_POINT ( 'NONE',  ( -5.571433138827826426, 0.000000000000000000, -10.72973591378220526 ) ) ;
#6222=CARTESIAN_POINT ( 'NONE',  ( 0.000000000000000000, 3.000000000000000000, 0.000000000000000000 ) ) ;
#6224=ORIENTED_EDGE ( 'NONE', *, *, #6021, .F. ) ;
#6225=CARTESIAN_POINT ( 'NONE',  ( 0.000000000000000000, 3.000000000000000000, 0.000000000000000000 ) ) ;
#6227=VECTOR ( 'NONE', #9145, 1000.000000000000000 ) ;
#6230=AXIS2_PLACEMENT_3D ( 'NONE', #4138, #7384, #9171 ) ;
#6233=VERTEX_POINT ( 'NONE', #11137 ) ;
#6241=ORIENTED_EDGE ( 'NONE', *, *, #13248, .F. ) ;
#6244=EDGE_CURVE ( 'NONE', #10564, #1235, #12991, .T. ) ;
#6247=DIRECTION ( 'NONE',  ( 0.000000000000000000, 0.000000000000000000, -1.000000000000000000 ) ) ;
#6272=ORIENTED_EDGE ( 'NONE', *, *, #8085, .T. ) ;
#6287=DIRECTION ( 'NONE',  ( 0.000000000000000000, 1.000000000000000000, 0.000000000000000000 ) ) ;
#6291=ORIENTED_EDGE ( 'NONE', *, *, #3722, .T. ) ;
#6292=CARTESIAN_POINT ( 'NONE',  ( -14.16466328168009881, 0.000000000000000000, 1.557181465540760534 ) ) ;
#6297=LINE ( 'NONE', #12314, #1634 ) ;
#6300=CARTESIAN_POINT ( 'NONE',  ( -11.48836750521723893, 0.000000000000000000, 8.430890348300625448 ) ) ;
#6302=B_SPLINE_CURVE_WITH_KNOTS ( 'NONE', 3,
 ( #7059, #2785, #8148, #5818 ),
 .UNSPECIFIED., .F., .F.,
 ( 4, 4 ),
 ( 0.1547128134717859205, 1.000000000000000000 ),
 .UNSPECIFIED. ) ;
#6304=CARTESIAN_POINT ( 'NONE',  ( -5.170206418547586225, 0.000000000000000000, 13.27898586450069907 ) ) ;
#6311=VERTEX_POINT ( 'NONE', #3682 ) ;
#6312=DIRECTION ( 'NONE',  ( 0.000000000000000000, 0.000000000000000000, 1.000000000000000000 ) ) ;
#6316=CARTESIAN_POINT ( 'NONE',  ( 13.27898586450069907, 3.000000000000000000, 5.170206418547587113 ) ) ;
#6327=EDGE_CURVE ( 'NONE', #3598, #7043, #9871, .T. ) ;
#6328=ORIENTED_EDGE ( 'NONE', *, *, #1453, .T. ) ;
#6329=B_SPLINE_SURFACE_WITH_KNOTS ( 'NONE', 3, 1, ( 
 ( #800, #7134 ),
 ( #12378, #6991 ),
 ( #651, #13465 ),
 ( #1756, #12091 ) ),
 .UNSPECIFIED., .F., .F., .F.,
 ( 4, 4 ),
 ( 2, 2 ),
 ( 0.1547128134717859205, 1.000000000000000000 ),
 ( 0.000000000000000000, 1.000000000000000000 ),
 .UNSPECIFIED. ) ;
#6330=CARTESIAN_POINT ( 'NONE',  ( -11.52666717836884125, 3.000000000000000000, -3.647470871583627705 ) ) ;
#6332=CARTESIAN_POINT ( 'NONE',  ( 3.647470871583629926, 0.000000000000000000, -11.52666717836884125 ) ) ;
#6343=ORIENTED_EDGE ( 'NONE', *, *, #5163, .T. ) ;
#6348=DIRECTION ( 'NONE',  ( 0.000000000000000000, 1.000000000000000000, 0.000000000000000000 ) ) ;
#6351=CARTESIAN_POINT ( 'NONE',  ( -2.161962830978702677, 3.000000000000000000, 14.08504230442587435 ) ) ;
#6358=CARTESIAN_POINT ( 'NONE',  ( -8.922136023539609440, 3.000000000000000000, 8.158651161643900807 ) ) ;
#6360=VERTEX_POINT ( 'NONE', #11477 ) ;
#6361=B_SPLINE_CURVE_WITH_KNOTS ( 'NONE', 3,
 ( #1128, #9531, #8418, #4024 ),
 .UNSPECIFIED., .F., .F.,
 ( 4, 4 ),
 ( 0.1547128134717859205, 1.000000000000000000 ),
 .UNSPECIFIED. ) ;
#6362=ORIENTED_EDGE ( 'NONE', *, *, #2194, .F. ) ;
#6363=AXIS2_PLACEMENT_3D ( 'NONE', #13422, #883, #10178 ) ;
#6369=CARTESIAN_POINT ( 'NONE',  ( 8.158551673544282679, 3.000000000000000000, -8.922226997226884393 ) ) ;
#6370=CIRCLE ( 'NONE', #230, 14.25000000000000178 ) ;
#6372=ORIENTED_EDGE ( 'NONE', *, *, #13578, .F. ) ;
#6373=CARTESIAN_POINT ( 'NONE',  ( 9.600126836553261711, 0.000000000000000000, 8.482622935103766082 ) ) ;
#6377=ADVANCED_FACE ( 'NONE', ( #7215 ), #1900, .F. ) ;
#6378=DIRECTION ( 'NONE',  ( 0.000000000000000000, 0.000000000000000000, -1.000000000000000000 ) ) ;
#6380=LINE ( 'NONE', #9484, #11675 ) ;
#6384=VECTOR ( 'NONE', #5016, 1000.000000000000000 ) ;
#6397=AXIS2_PLACEMENT_3D ( 'NONE', #10318, #2877, #13361 ) ;
#6398=DIRECTION ( 'NONE',  ( 0.000000000000000000, 0.000000000000000000, 1.000000000000000000 ) ) ;
#6399=DIRECTION ( 'NONE',  ( -0.000000000000000000, -1.000000000000000000, -0.000000000000000000 ) ) ;
#6404=CARTESIAN_POINT ( 'NONE',  ( -13.50994833511691340, 3.000000000000000000, -1.105736515254444052 ) ) ;
#6408=CYLINDRICAL_SURFACE ( 'NONE', #2688, 12.08999999999737440 ) ;
#6418=DIRECTION ( 'NONE',  ( -0.000000000000000000, -1.000000000000000000, -0.000000000000000000 ) ) ;
#6420=EDGE_CURVE ( 'NONE', #5900, #3087, #5969, .T. ) ;
#6421=CARTESIAN_POINT ( 'NONE',  ( 2.546103534247748712, 0.000000000000000000, -12.55526518755974585 ) ) ;
#6422=EDGE_CURVE ( 'NONE', #12936, #2347, #3603, .T. ) ;
#6424=DIRECTION ( 'NONE',  ( 0.000000000000000000, 0.000000000000000000, -1.000000000000000000 ) ) ;
#6435=EDGE_CURVE ( 'NONE', #97, #1924, #4311, .T. ) ;
#6438=CARTESIAN_POINT ( 'NONE',  ( -10.67828022838850721, 0.000000000000000000, 7.077546079049267469 ) ) ;
#6448=CARTESIAN_POINT ( 'NONE',  ( 11.11702303352196708, 3.000000000000000000, 8.914835885878218846 ) ) ;
#6459=CARTESIAN_POINT ( 'NONE',  ( -8.760376775873710997, 0.000000000000000000, 10.34346111134700941 ) ) ;
#6463=CIRCLE ( 'NONE', #7564, 12.08999999999737440 ) ;
#6464=ORIENTED_EDGE ( 'NONE', *, *, #6518, .T. ) ;
#6467=CARTESIAN_POINT ( 'NONE',  ( 8.914835885878220623, 3.000000000000000000, -11.11702303352196708 ) ) ;
#6468=ORIENTED_EDGE ( 'NONE', *, *, #4889, .T. ) ;
#6471=SURFACE_STYLE_FILL_AREA ( #6197 ) ;
#6478=EDGE_LOOP ( 'NONE', ( #6291, #6579, #9389, #2802 ) ) ;
#6479=CYLINDRICAL_SURFACE ( 'NONE', #4248, 14.25000000000000178 ) ;
#6494=CARTESIAN_POINT ( 'NONE',  ( 8.914835885878215294, 3.000000000000000000, 11.11702303352197418 ) ) ;
#6496=LINE ( 'NONE', #8071, #5529 ) ;
#6502=EDGE_CURVE ( 'NONE', #8926, #9781, #9912, .T. ) ;
#6503=ORIENTED_EDGE ( 'NONE', *, *, #2669, .T. ) ;
#6509=CARTESIAN_POINT ( 'NONE',  ( 3.647470871583629926, 3.000000000000000000, -11.52666717836884125 ) ) ;
#6513=DIRECTION ( 'NONE',  ( 0.000000000000000000, 1.000000000000000000, 0.000000000000000000 ) ) ;
#6518=EDGE_CURVE ( 'NONE', #313, #9964, #10, .T. ) ;
#6519=VERTEX_POINT ( 'NONE', #4438 ) ;
#6524=CARTESIAN_POINT ( 'NONE',  ( -13.27898586450070084, 0.000000000000000000, -5.170206418547588001 ) ) ;
#6529=CARTESIAN_POINT ( 'NONE',  ( 1.557181465540672161, 0.000000000000000000, -14.16466328168010591 ) ) ;
#6530=ORIENTED_EDGE ( 'NONE', *, *, #4572, .F. ) ;
#6531=EDGE_LOOP ( 'NONE', ( #7567, #8424, #5079, #2909 ) ) ;
#6532=ORIENTED_EDGE ( 'NONE', *, *, #8436, .T. ) ;
#6535=ORIENTED_EDGE ( 'NONE', *, *, #11243, .F. ) ;
#6538=B_SPLINE_CURVE_WITH_KNOTS ( 'NONE', 3,
 ( #9834, #6677, #10880, #4604 ),
 .UNSPECIFIED., .F., .F.,
 ( 4, 4 ),
 ( 0.1547128134717859205, 1.000000000000000000 ),
 .UNSPECIFIED. ) ;
#6540=B_SPLINE_SURFACE_WITH_KNOTS ( 'NONE', 3, 1, ( 
 ( #3748, #7750 ),
 ( #7953, #8712 ),
 ( #12929, #2726 ),
 ( #11966, #1427 ) ),
 .UNSPECIFIED., .F., .F., .F.,
 ( 4, 4 ),
 ( 2, 2 ),
 ( 0.1547128134717859205, 1.000000000000000000 ),
 ( 0.000000000000000000, 1.000000000000000000 ),
 .UNSPECIFIED. ) ;
#6541=CARTESIAN_POINT ( 'NONE',  ( 4.056222772158357692, 3.000000000000000000, -12.16218796965919680 ) ) ;
#6547=( NAMED_UNIT ( * ) PLANE_ANGLE_UNIT ( ) SI_UNIT ( $, .RADIAN. ) );
#6553=ORIENTED_EDGE ( 'NONE', *, *, #9313, .T. ) ;
#6554=DIRECTION ( 'NONE',  ( 0.000000000000000000, 0.000000000000000000, -1.000000000000000000 ) ) ;
#6558=EDGE_CURVE ( 'NONE', #523, #7235, #7070, .T. ) ;
#6561=LINE ( 'NONE', #8547, #11556 ) ;
#6562=ORIENTED_EDGE ( 'NONE', *, *, #2447, .T. ) ;
#6564=ORIENTED_EDGE ( 'NONE', *, *, #11661, .F. ) ;
#6565=EDGE_LOOP ( 'NONE', ( #5954, #6012, #6751, #1797 ) ) ;
#6568=CARTESIAN_POINT ( 'NONE',  ( 0.000000000000000000, 3.000000000000000000, 0.000000000000000000 ) ) ;
#6575=EDGE_CURVE ( 'NONE', #10694, #11321, #9042, .T. ) ;
#6579=ORIENTED_EDGE ( 'NONE', *, *, #5222, .F. ) ;
#6582=CARTESIAN_POINT ( 'NONE',  ( -11.46814821560793440, 3.000000000000000000, 5.731782959214994477 ) ) ;
#6583=CARTESIAN_POINT ( 'NONE',  ( -13.04554897075799680, 3.000000000000000000, -5.733772933379471581 ) ) ;
#6585=DIRECTION ( 'NONE',  ( 0.000000000000000000, 0.000000000000000000, 1.000000000000000000 ) ) ;
#6590=CARTESIAN_POINT ( 'NONE',  ( 3.647599401157691101, 0.000000000000000000, 11.52662650599084238 ) ) ;
#6591=VERTEX_POINT ( 'NONE', #1757 ) ;
#6597=CIRCLE ( 'NONE', #1539, 12.08999999999737440 ) ;
#6605=AXIS2_PLACEMENT_3D ( 'NONE', #8904, #1618, #13047 ) ;
#6607=B_SPLINE_SURFACE_WITH_KNOTS ( 'NONE', 3, 1, ( 
 ( #8636, #11822 ),
 ( #10778, #6373 ),
 ( #3336, #8437 ),
 ( #10659, #7620 ) ),
 .UNSPECIFIED., .F., .F., .F.,
 ( 4, 4 ),
 ( 2, 2 ),
 ( 0.1547128134717859205, 1.000000000000000000 ),
 ( 0.000000000000000000, 1.000000000000000000 ),
 .UNSPECIFIED. ) ;
#6609=CYLINDRICAL_SURFACE ( 'NONE', #10008, 12.08999999999737440 ) ;
#6613=EDGE_LOOP ( 'NONE', ( #6863, #12711, #11373, #9162 ) ) ;
#6616=VERTEX_POINT ( 'NONE', #8827 ) ;
#6619=AXIS2_PLACEMENT_3D ( 'NONE', #12269, #6058, #4953 ) ;
#6621=CARTESIAN_POINT ( 'NONE',  ( 0.000000000000000000, 0.000000000000000000, 0.000000000000000000 ) ) ;
#6630=ORIENTED_EDGE ( 'NONE', *, *, #6101, .T. ) ;
#6633=B_SPLINE_SURFACE_WITH_KNOTS ( 'NONE', 3, 1, ( 
 ( #12481, #71 ),
 ( #9561, #3019 ),
 ( #7226, #7487 ),
 ( #11691, #2182 ) ),
 .UNSPECIFIED., .F., .F., .F.,
 ( 4, 4 ),
 ( 2, 2 ),
 ( 0.000000000000000000, 0.8452273900860258760 ),
 ( 0.000000000000000000, 1.000000000000000000 ),
 .UNSPECIFIED. ) ;
#6639=LINE ( 'NONE', #2375, #9005 ) ;
#6640=CARTESIAN_POINT ( 'NONE',  ( -10.18979803820068675, 0.000000000000000000, 6.506620931068438196 ) ) ;
#6647=EDGE_CURVE ( 'NONE', #10019, #9707, #10082, .T. ) ;
#6648=EDGE_CURVE ( 'NONE', #8949, #97, #11259, .T. ) ;
#6658=CARTESIAN_POINT ( 'NONE',  ( 11.13895890373327724, 0.000000000000000000, -7.723663868796764476 ) ) ;
#6660=CARTESIAN_POINT ( 'NONE',  ( -5.571433138827826426, 3.000000000000000000, -10.72973591378220526 ) ) ;
#6662=ORIENTED_EDGE ( 'NONE', *, *, #12071, .T. ) ;
#6668=VERTEX_POINT ( 'NONE', #4920 ) ;
#6671=AXIS2_PLACEMENT_3D ( 'NONE', #689, #7780, #9078 ) ;
#6673=EDGE_CURVE ( 'NONE', #9781, #4442, #9193, .T. ) ;
#6677=CARTESIAN_POINT ( 'NONE',  ( -9.600126836553261711, 0.000000000000000000, -8.482622935103767858 ) ) ;
#6683=VERTEX_POINT ( 'NONE', #9937 ) ;
#6688=CARTESIAN_POINT ( 'NONE',  ( 0.000000000000000000, 0.000000000000000000, 0.000000000000000000 ) ) ;
#6692=ORIENTED_EDGE ( 'NONE', *, *, #6200, .T. ) ;
#6697=DIRECTION ( 'NONE',  ( -0.000000000000000000, -1.000000000000000000, -0.000000000000000000 ) ) ;
#6698=DIRECTION ( 'NONE',  ( 0.000000000000000000, 0.000000000000000000, -1.000000000000000000 ) ) ;
#6703=ORIENTED_EDGE ( 'NONE', *, *, #12040, .F. ) ;
#6706=CARTESIAN_POINT ( 'NONE',  ( 0.5398653231797245766, 3.000000000000000000, -12.07794044664754018 ) ) ;
#6708=AXIS2_PLACEMENT_3D ( 'NONE', #3590, #12907, #2362 ) ;
#6710=CYLINDRICAL_SURFACE ( 'NONE', #443, 14.25000000000000178 ) ;
#6717=ORIENTED_EDGE ( 'NONE', *, *, #1655, .F. ) ;
#6719=CARTESIAN_POINT ( 'NONE',  ( -8.158551673544284455, 0.000000000000000000, 8.922226997226891498 ) ) ;
#6724=CARTESIAN_POINT ( 'NONE',  ( 10.18979803820051622, 0.000000000000000000, -6.506620931068703761 ) ) ;
#6725=EDGE_CURVE ( 'NONE', #523, #4083, #7399, .T. ) ;
#6727=CARTESIAN_POINT ( 'NONE',  ( 12.46219022525837694, 3.000000000000000000, -4.344528055836598845 ) ) ;
#6731=VERTEX_POINT ( 'NONE', #2027 ) ;
#6736=CARTESIAN_POINT ( 'NONE',  ( 5.784789447945496654, 0.000000000000000000, -12.25836857253663581 ) ) ;
#6737=ADVANCED_FACE ( 'NONE', ( #5121 ), #10430, .T. ) ;
#6741=CARTESIAN_POINT ( 'NONE',  ( 5.784789447945496654, 3.000000000000000000, -12.25836857253663581 ) ) ;
#6742=CYLINDRICAL_SURFACE ( 'NONE', #11701, 14.24999999999999822 ) ;
#6747=EDGE_CURVE ( 'NONE', #1810, #9927, #8522, .T. ) ;
#6751=ORIENTED_EDGE ( 'NONE', *, *, #5721, .F. ) ;
#6754=CARTESIAN_POINT ( 'NONE',  ( 0.000000000000000000, 0.000000000000000000, 0.000000000000000000 ) ) ;
#6762=B_SPLINE_SURFACE_WITH_KNOTS ( 'NONE', 3, 1, ( 
 ( #9719, #7599 ),
 ( #7722, #6421 ),
 ( #4358, #2360 ),
 ( #11799, #9853 ) ),
 .UNSPECIFIED., .F., .F., .F.,
 ( 4, 4 ),
 ( 2, 2 ),
 ( 0.1547128134717859205, 1.000000000000000000 ),
 ( 0.000000000000000000, 1.000000000000000000 ),
 .UNSPECIFIED. ) ;
#6770=CARTESIAN_POINT ( 'NONE',  ( -8.504652361247167391, 3.000000000000000000, -9.593885948927674434 ) ) ;
#6779=ORIENTED_EDGE ( 'NONE', *, *, #6725, .T. ) ;
#6786=LINE ( 'NONE', #2729, #11234 ) ;
#6796=VECTOR ( 'NONE', #12808, 1000.000000000000000 ) ;
#6797=CARTESIAN_POINT ( 'NONE',  ( 0.000000000000000000, 3.000000000000000000, 0.000000000000000000 ) ) ;
#6800=LINE ( 'NONE', #10698, #13441 ) ;
#6810=EDGE_LOOP ( 'NONE', ( #6468, #10111, #10297, #6979 ) ) ;
#6812=EDGE_CURVE ( 'NONE', #11589, #3853, #11335, .T. ) ;
#6814=ORIENTED_EDGE ( 'NONE', *, *, #8337, .T. ) ;
#6816=CARTESIAN_POINT ( 'NONE',  ( 11.11702303352196708, 0.000000000000000000, 8.914835885878218846 ) ) ;
#6818=AXIS2_PLACEMENT_3D ( 'NONE', #2198, #6399, #8527 ) ;
#6821=CIRCLE ( 'NONE', #2201, 12.08999999999737085 ) ;
#6822=CARTESIAN_POINT ( 'NONE',  ( -12.78643498603817896, 0.000000000000000000, 0.7901945867173603144 ) ) ;
#6823=CARTESIAN_POINT ( 'NONE',  ( 8.760376775873721655, 3.000000000000000000, -10.34346111134700585 ) ) ;
#6825=ORIENTED_EDGE ( 'NONE', *, *, #5889, .F. ) ;
#6832=AXIS2_PLACEMENT_3D ( 'NONE', #9071, #11423, #13290 ) ;
#6840=CARTESIAN_POINT ( 'NONE',  ( -10.72973591378220348, 0.000000000000000000, 5.571433138827830867 ) ) ;
#6842=CARTESIAN_POINT ( 'NONE',  ( -14.16466328168010769, 3.000000000000000000, -1.557181465540673271 ) ) ;
#6847=CARTESIAN_POINT ( 'NONE',  ( 10.18979803820052155, 0.000000000000000000, -6.506620931068708202 ) ) ;
#6848=PLANE ( 'NONE',  #13265 ) ;
#6852=VECTOR ( 'NONE', #1903, 1000.000000000000000 ) ;
#6854=CARTESIAN_POINT ( 'NONE',  ( 12.25282671965375592, 0.000000000000000000, -5.797378255456012930 ) ) ;
#6856=CARTESIAN_POINT ( 'NONE',  ( -8.158651161643904359, 0.000000000000000000, -8.922136023539605887 ) ) ;
#6858=CARTESIAN_POINT ( 'NONE',  ( -12.56087513340552242, 3.000000000000000000, 2.568302020731519253 ) ) ;
#6860=AXIS2_PLACEMENT_3D ( 'NONE', #2377, #442, #5407 ) ;
#6863=ORIENTED_EDGE ( 'NONE', *, *, #11909, .T. ) ;
#6864=EDGE_CURVE ( 'NONE', #7415, #205, #13149, .T. ) ;
#6865=EDGE_LOOP ( 'NONE', ( #4689, #1591, #8852, #6562 ) ) ;
#6869=ORIENTED_EDGE ( 'NONE', *, *, #6327, .T. ) ;
#6872=AXIS2_PLACEMENT_3D ( 'NONE', #9660, #7726, #1471 ) ;
#6873=DIRECTION ( 'NONE',  ( 0.000000000000000000, 0.000000000000000000, 1.000000000000000000 ) ) ;
#6886=CARTESIAN_POINT ( 'NONE',  ( -7.065816209474154341, 3.000000000000000000, 10.69794375946289833 ) ) ;
#6887=ORIENTED_EDGE ( 'NONE', *, *, #10469, .F. ) ;
#6892=AXIS2_PLACEMENT_3D ( 'NONE', #6150, #8483, #10353 ) ;
#6898=CARTESIAN_POINT ( 'NONE',  ( 0.000000000000000000, 0.000000000000000000, 0.000000000000000000 ) ) ;
#6899=EDGE_CURVE ( 'NONE', #3720, #11537, #7401, .T. ) ;
#6902=ORIENTED_EDGE ( 'NONE', *, *, #8337, .F. ) ;
#6904=AXIS2_PLACEMENT_3D ( 'NONE', #9918, #5794, #1598 ) ;
#6911=CARTESIAN_POINT ( 'NONE',  ( 0.000000000000000000, 3.000000000000000000, 0.000000000000000000 ) ) ;
#6912=B_SPLINE_CURVE_WITH_KNOTS ( 'NONE', 3,
 ( #6968, #13439, #9013, #3992 ),
 .UNSPECIFIED., .F., .F.,
 ( 4, 4 ),
 ( 0.000000000000000000, 0.8452273900860258760 ),
 .UNSPECIFIED. ) ;
#6917=EDGE_CURVE ( 'NONE', #9840, #1800, #10023, .T. ) ;
#6918=DIRECTION ( 'NONE',  ( 0.000000000000000000, 1.000000000000000000, 0.000000000000000000 ) ) ;
#6920=EDGE_CURVE ( 'NONE', #3087, #9002, #5413, .T. ) ;
#6921=LINE ( 'NONE', #9185, #2264 ) ;
#6922=CARTESIAN_POINT ( 'NONE',  ( 31.00000000000000000, 3.000000000000000000, 3.999999998926329514 ) ) ;
#6923=EDGE_LOOP ( 'NONE', ( #988, #982, #9557, #11719 ) ) ;
#6925=ORIENTED_EDGE ( 'NONE', *, *, #11069, .F. ) ;
#6926=ADVANCED_FACE ( 'NONE', ( #9528 ), #109, .T. ) ;
#6928=VECTOR ( 'NONE', #5248, 1000.000000000000000 ) ;
#6930=CARTESIAN_POINT ( 'NONE',  ( 5.731782959214990036, 0.000000000000000000, 11.46814821560793618 ) ) ;
#6932=CARTESIAN_POINT ( 'NONE',  ( -10.18987059060247624, 3.000000000000000000, -6.506507307819711095 ) ) ;
#6933=B_SPLINE_CURVE_WITH_KNOTS ( 'NONE', 3,
 ( #9623, #7426, #6459, #335 ),
 .UNSPECIFIED., .F., .F.,
 ( 4, 4 ),
 ( 0.1547128134717859205, 1.000000000000000000 ),
 .UNSPECIFIED. ) ;
#6936=LINE ( 'NONE', #2796, #5286 ) ;
#6938=CARTESIAN_POINT ( 'NONE',  ( 13.27898586450067242, 3.000000000000000000, -5.170206418547655502 ) ) ;
#6945=ORIENTED_EDGE ( 'NONE', *, *, #303, .T. ) ;
#6950=CARTESIAN_POINT ( 'NONE',  ( -2.568302020731516588, 3.000000000000000000, -12.56087513340552242 ) ) ;
#6952=EDGE_CURVE ( 'NONE', #1933, #9046, #11175, .T. ) ;
#6955=EDGE_CURVE ( 'NONE', #1864, #10087, #6496, .T. ) ;
#6956=CARTESIAN_POINT ( 'NONE',  ( 5.571313494980132397, 3.000000000000000000, -10.72979803820131472 ) ) ;
#6958=CARTESIAN_POINT ( 'NONE',  ( 2.568302020731520141, 0.000000000000000000, 12.56087513340552420 ) ) ;
#6968=CARTESIAN_POINT ( 'NONE',  ( -11.48836750521728689, 0.000000000000000000, -8.430890348300561499 ) ) ;
#6974=CARTESIAN_POINT ( 'NONE',  ( -1.557181465540760534, 0.000000000000000000, -14.16466328168009703 ) ) ;
#6979=ORIENTED_EDGE ( 'NONE', *, *, #3044, .T. ) ;
#6980=CARTESIAN_POINT ( 'NONE',  ( -1.105736515254454044, 3.000000000000000000, 13.50994833511691340 ) ) ;
#6982=EDGE_CURVE ( 'NONE', #9461, #13528, #7867, .T. ) ;
#6990=B_SPLINE_SURFACE_WITH_KNOTS ( 'NONE', 3, 1, ( 
 ( #5974, #1855 ),
 ( #2743, #3845 ),
 ( #6950, #6055 ),
 ( #1652, #5844 ) ),
 .UNSPECIFIED., .F., .F., .F.,
 ( 4, 4 ),
 ( 2, 2 ),
 ( 0.000000000000000000, 0.8452273900860258760 ),
 ( 0.000000000000000000, 1.000000000000000000 ),
 .UNSPECIFIED. ) ;
#6991=CARTESIAN_POINT ( 'NONE',  ( -7.077546079049271910, 0.000000000000000000, -10.67828022838850544 ) ) ;
#6995=ORIENTED_EDGE ( 'NONE', *, *, #7677, .T. ) ;
#6999=EDGE_CURVE ( 'NONE', #7580, #1090, #4763, .T. ) ;
#7001=CARTESIAN_POINT ( 'NONE',  ( -8.760376775873710997, 3.000000000000000000, 10.34346111134700941 ) ) ;
#7005=FACE_OUTER_BOUND ( 'NONE', #7811, .T. ) ;
#7009=CARTESIAN_POINT ( 'NONE',  ( -1.105736515254454044, 0.000000000000000000, 13.50994833511691340 ) ) ;
#7019=FACE_OUTER_BOUND ( 'NONE', #4977, .T. ) ;
#7026=ORIENTED_EDGE ( 'NONE', *, *, #1991, .F. ) ;
#7027=EDGE_LOOP ( 'NONE', ( #6662, #12275, #12294, #3298 ) ) ;
#7029=ADVANCED_FACE ( 'NONE', ( #3654 ), #2565, .T. ) ;
#7033=ORIENTED_EDGE ( 'NONE', *, *, #690, .T. ) ;
#7039=AXIS2_PLACEMENT_3D ( 'NONE', #7498, #2340, #7439 ) ;
#7041=ORIENTED_EDGE ( 'NONE', *, *, #7746, .T. ) ;
#7043=VERTEX_POINT ( 'NONE', #11170 ) ;
#7048=ORIENTED_EDGE ( 'NONE', *, *, #5723, .F. ) ;
#7052=CARTESIAN_POINT ( 'NONE',  ( 9.593885948927676210, 0.000000000000000000, -8.504652361247169168 ) ) ;
#7053=CARTESIAN_POINT ( 'NONE',  ( -8.914835885878284572, 0.000000000000000000, -11.11702303352191379 ) ) ;
#7055=DIRECTION ( 'NONE',  ( 0.000000000000000000, 1.000000000000000000, 0.000000000000000000 ) ) ;
#7057=LINE ( 'NONE', #1692, #2662 ) ;
#7058=DIRECTION ( 'NONE',  ( -0.000000000000000000, -1.000000000000000000, -0.000000000000000000 ) ) ;
#7059=CARTESIAN_POINT ( 'NONE',  ( -0.5400000000007666445, 0.000000000000000000, -12.07793442604883793 ) ) ;
#7061=VECTOR ( 'NONE', #10592, 1000.000000000000000 ) ;
#7068=DIRECTION ( 'NONE',  ( -1.000000000000000000, 0.000000000000000000, 1.370446048119726253E-16 ) ) ;
#7070=CIRCLE ( 'NONE', #11683, 12.08999999999737440 ) ;
#7081=DIRECTION ( 'NONE',  ( -0.000000000000000000, -1.000000000000000000, -0.000000000000000000 ) ) ;
#7083=ORIENTED_EDGE ( 'NONE', *, *, #753, .F. ) ;
#7090=CARTESIAN_POINT ( 'NONE',  ( -8.922136023539609440, 0.000000000000000000, 8.158651161643900807 ) ) ;
#7101=EDGE_CURVE ( 'NONE', #1063, #2645, #3996, .T. ) ;
#7102=ORIENTED_EDGE ( 'NONE', *, *, #7677, .F. ) ;
#7105=EDGE_CURVE ( 'NONE', #3224, #12936, #11314, .T. ) ;
#7107=B_SPLINE_SURFACE_WITH_KNOTS ( 'NONE', 3, 1, ( 
 ( #12214, #3587 ),
 ( #11025, #4826 ),
 ( #9017, #1596 ),
 ( #571, #13234 ) ),
 .UNSPECIFIED., .F., .F., .F.,
 ( 4, 4 ),
 ( 2, 2 ),
 ( 0.1547128134717859205, 1.000000000000000000 ),
 ( 0.000000000000000000, 1.000000000000000000 ),
 .UNSPECIFIED. ) ;
#7112=DIRECTION ( 'NONE',  ( 0.000000000000000000, 0.000000000000000000, 1.000000000000000000 ) ) ;
#7114=AXIS2_PLACEMENT_3D ( 'NONE', #12968, #9858, #12708 ) ;
#7121=EDGE_LOOP ( 'NONE', ( #13588, #3301, #8455, #12646 ) ) ;
#7134=CARTESIAN_POINT ( 'NONE',  ( -6.506620931068715308, 0.000000000000000000, -10.18979803820051799 ) ) ;
#7139=CARTESIAN_POINT ( 'NONE',  ( 13.04554897075796838, 0.000000000000000000, -5.733772933379540859 ) ) ;
#7141=ORIENTED_EDGE ( 'NONE', *, *, #1203, .F. ) ;
#7142=VERTEX_POINT ( 'NONE', #5101 ) ;
#7147=AXIS2_PLACEMENT_3D ( 'NONE', #8984, #13199, #12183 ) ;
#7148=CARTESIAN_POINT ( 'NONE',  ( 10.72979803820131472, 0.000000000000000000, 5.571313494980131509 ) ) ;
#7154=DIRECTION ( 'NONE',  ( 0.000000000000000000, 1.000000000000000000, 0.000000000000000000 ) ) ;
#7168=CARTESIAN_POINT ( 'NONE',  ( 10.72979803820131472, 3.000000000000000000, 5.571313494980131509 ) ) ;
#7169=CARTESIAN_POINT ( 'NONE',  ( 13.27898586450067420, 0.000000000000000000, 5.170206418547648397 ) ) ;
#7173=ORIENTED_EDGE ( 'NONE', *, *, #4492, .T. ) ;
#7174=CARTESIAN_POINT ( 'NONE',  ( 0.000000000000000000, 0.000000000000000000, -12.08999999999737440 ) ) ;
#7183=CARTESIAN_POINT ( 'NONE',  ( 13.04554897075798081, 3.000000000000000000, -5.733772933379503556 ) ) ;
#7201=EDGE_CURVE ( 'NONE', #2104, #13127, #261, .T. ) ;
#7202=FACE_OUTER_BOUND ( 'NONE', #12516, .T. ) ;
#7213=CARTESIAN_POINT ( 'NONE',  ( -13.04554897075799680, 3.000000000000000000, -5.733772933379471581 ) ) ;
#7215=FACE_OUTER_BOUND ( 'NONE', #4300, .T. ) ;
#7218=VERTEX_POINT ( 'NONE', #11645 ) ;
#7219=CARTESIAN_POINT ( 'NONE',  ( 12.03251085770905959, 0.000000000000000000, 3.999999998926332179 ) ) ;
#7222=ORIENTED_EDGE ( 'NONE', *, *, #4993, .F. ) ;
#7223=DIRECTION ( 'NONE',  ( -0.000000000000000000, -1.000000000000000000, -0.000000000000000000 ) ) ;
#7225=CARTESIAN_POINT ( 'NONE',  ( -14.08504230442587790, 0.000000000000000000, -2.161962830978695571 ) ) ;
#7226=CARTESIAN_POINT ( 'NONE',  ( 2.568302020731520141, 3.000000000000000000, 12.56087513340552420 ) ) ;
#7229=CARTESIAN_POINT ( 'NONE',  ( 12.25836857253663581, 3.000000000000000000, 5.784789447945493990 ) ) ;
#7230=CARTESIAN_POINT ( 'NONE',  ( -11.52666717836884125, 3.000000000000000000, -3.647470871583627705 ) ) ;
#7232=ORIENTED_EDGE ( 'NONE', *, *, #6558, .F. ) ;
#7233=UNCERTAINTY_MEASURE_WITH_UNIT (LENGTH_MEASURE( 1.000000000000000082E-05 ), #12750, 'distance_accuracy_value', 'NONE');
#7235=VERTEX_POINT ( 'NONE', #4344 ) ;
#7236=CARTESIAN_POINT ( 'NONE',  ( 0.000000000000000000, 3.000000000000000000, 0.000000000000000000 ) ) ;
#7239=SHAPE_REPRESENTATION_RELATIONSHIP ( 'NONE' , 'NONE' ,  #2323, #7847 ) ;
#7241=CARTESIAN_POINT ( 'NONE',  ( 10.18987059060247269, 3.000000000000000000, 6.506507307819714647 ) ) ;
#7244=CARTESIAN_POINT ( 'NONE',  ( 31.00000000000000000, 3.000000000000000000, -4.000000001073670930 ) ) ;
#7252=B_SPLINE_CURVE_WITH_KNOTS ( 'NONE', 3,
 ( #11491, #13496, #4050, #11571 ),
 .UNSPECIFIED., .F., .F.,
 ( 4, 4 ),
 ( 0.000000000000000000, 0.8452273900860258760 ),
 .UNSPECIFIED. ) ;
#7258=AXIS2_PLACEMENT_3D ( 'NONE', #3090, #7303, #11504 ) ;
#7259=LINE ( 'NONE', #6093, #7915 ) ;
#7262=CARTESIAN_POINT ( 'NONE',  ( 3.647599401157688437, 3.000000000000000000, 11.52662650599083882 ) ) ;
#7265=B_SPLINE_CURVE_WITH_KNOTS ( 'NONE', 3,
 ( #5404, #7278, #9609, #3128 ),
 .UNSPECIFIED., .F., .F.,
 ( 4, 4 ),
 ( 0.000000000000000000, 0.8452273900860258760 ),
 .UNSPECIFIED. ) ;
#7270=VERTEX_POINT ( 'NONE', #10612 ) ;
#7271=EDGE_CURVE ( 'NONE', #10338, #9457, #13449, .T. ) ;
#7272=EDGE_CURVE ( 'NONE', #1406, #4083, #12310, .T. ) ;
#7275=CARTESIAN_POINT ( 'NONE',  ( 0.000000000000000000, 3.000000000000000000, 0.000000000000000000 ) ) ;
#7278=CARTESIAN_POINT ( 'NONE',  ( 8.771102293099069414, 3.000000000000000000, 10.33484986938308303 ) ) ;
#7283=ORIENTED_EDGE ( 'NONE', *, *, #13300, .T. ) ;
#7285=CARTESIAN_POINT ( 'NONE',  ( 11.46847481510586775, 0.000000000000000000, 5.708888906988908829 ) ) ;
#7295=AXIS2_PLACEMENT_3D ( 'NONE', #10307, #873, #13196 ) ;
#7301=ORIENTED_EDGE ( 'NONE', *, *, #3694, .T. ) ;
#7303=DIRECTION ( 'NONE',  ( 0.000000000000000000, 1.000000000000000000, 0.000000000000000000 ) ) ;
#7306=FACE_OUTER_BOUND ( 'NONE', #7714, .T. ) ;
#7309=CARTESIAN_POINT ( 'NONE',  ( -4.577511697546077230, 0.000000000000000000, -12.75843939030334795 ) ) ;
#7310=VERTEX_POINT ( 'NONE', #90 ) ;
#7313=ORIENTED_EDGE ( 'NONE', *, *, #8613, .T. ) ;
#7324=EDGE_CURVE ( 'NONE', #13528, #7270, #3170, .T. ) ;
#7325=CARTESIAN_POINT ( 'NONE',  ( -5.708888906988910605, 0.000000000000000000, 11.46847481510586597 ) ) ;
#7330=LINE ( 'NONE', #5200, #9296 ) ;
#7334=CIRCLE ( 'NONE', #9953, 14.25000000000000178 ) ;
#7343=CARTESIAN_POINT ( 'NONE',  ( -10.18979803820052155, 0.000000000000000000, 6.506620931068709091 ) ) ;
#7349=CARTESIAN_POINT ( 'NONE',  ( -10.18987059060247624, 3.000000000000000000, -6.506507307819711095 ) ) ;
#7350=AXIS2_PLACEMENT_3D ( 'NONE', #8030, #8095, #11471 ) ;
#7354=CARTESIAN_POINT ( 'NONE',  ( 8.914835885878220623, 0.000000000000000000, -11.11702303352196708 ) ) ;
#7360=VECTOR ( 'NONE', #1765, 1000.000000000000000 ) ;
#7365=VECTOR ( 'NONE', #10755, 1000.000000000000000 ) ;
#7367=ORIENTED_EDGE ( 'NONE', *, *, #5007, .F. ) ;
#7368=ORIENTED_EDGE ( 'NONE', *, *, #7843, .F. ) ;
#7369=ORIENTED_EDGE ( 'NONE', *, *, #8036, .T. ) ;
#7374=ADVANCED_FACE ( 'NONE', ( #4542 ), #7777, .T. ) ;
#7378=CARTESIAN_POINT ( 'NONE',  ( -12.75843939030334795, 3.000000000000000000, 4.577511697546079006 ) ) ;
#7384=DIRECTION ( 'NONE',  ( 0.000000000000000000, 1.000000000000000000, 0.000000000000000000 ) ) ;
#7385=ORIENTED_EDGE ( 'NONE', *, *, #6518, .F. ) ;
#7387=ORIENTED_EDGE ( 'NONE', *, *, #6673, .T. ) ;
#7394=DIRECTION ( 'NONE',  ( 0.000000000000000000, 0.000000000000000000, 1.000000000000000000 ) ) ;
#7396=FACE_OUTER_BOUND ( 'NONE', #10719, .T. ) ;
#7397=LINE ( 'NONE', #11332, #964 ) ;
#7399=LINE ( 'NONE', #2994, #10586 ) ;
#7400=CARTESIAN_POINT ( 'NONE',  ( 10.18987059060247269, 0.000000000000000000, 6.506507307819714647 ) ) ;
#7401=B_SPLINE_CURVE_WITH_KNOTS ( 'NONE', 3,
 ( #2422, #7461, #5517, #8484 ),
 .UNSPECIFIED., .F., .F.,
 ( 4, 4 ),
 ( 0.000000000000000000, 0.8452273900860258760 ),
 .UNSPECIFIED. ) ;
#7404=ORIENTED_EDGE ( 'NONE', *, *, #8503, .F. ) ;
#7408=VERTEX_POINT ( 'NONE', #3699 ) ;
#7409=CARTESIAN_POINT ( 'NONE',  ( -5.571313494980134173, 3.000000000000000000, 10.72979803820131295 ) ) ;
#7410=LINE ( 'NONE', #6509, #5789 ) ;
#7415=VERTEX_POINT ( 'NONE', #620 ) ;
#7421=DIRECTION ( 'NONE',  ( -0.000000000000000000, -1.000000000000000000, -0.000000000000000000 ) ) ;
#7423=CARTESIAN_POINT ( 'NONE',  ( 0.000000000000000000, 3.000000000000000000, 0.000000000000000000 ) ) ;
#7424=CARTESIAN_POINT ( 'NONE',  ( 5.170206418547604876, 3.000000000000000000, -13.27898586450069196 ) ) ;
#7426=CARTESIAN_POINT ( 'NONE',  ( -8.482622935103766082, 0.000000000000000000, 9.600126836553263487 ) ) ;
#7430=ADVANCED_FACE ( 'NONE', ( #12947 ), #6742, .T. ) ;
#7436=ADVANCED_FACE ( 'NONE', ( #5775 ), #2606, .T. ) ;
#7439=DIRECTION ( 'NONE',  ( 0.000000000000000000, 0.000000000000000000, 1.000000000000000000 ) ) ;
#7440=CARTESIAN_POINT ( 'NONE',  ( 5.733772933379474246, 3.000000000000000000, -13.04554897075799502 ) ) ;
#7446=CARTESIAN_POINT ( 'NONE',  ( -12.07794044664754018, 3.000000000000000000, -0.5398653231797256868 ) ) ;
#7447=ORIENTED_EDGE ( 'NONE', *, *, #10821, .F. ) ;
#7452=DIRECTION ( 'NONE',  ( 0.000000000000000000, 1.000000000000000000, 0.000000000000000000 ) ) ;
#7454=ADVANCED_FACE ( 'NONE', ( #11915 ), #4444, .F. ) ;
#7458=CARTESIAN_POINT ( 'NONE',  ( -10.72979803820123479, 3.000000000000000000, -5.571313494980285164 ) ) ;
#7459=CARTESIAN_POINT ( 'NONE',  ( -12.76342233970728124, 3.000000000000000000, -4.564691384634500970 ) ) ;
#7461=CARTESIAN_POINT ( 'NONE',  ( -12.25282671965375236, 0.000000000000000000, 5.797378255456025364 ) ) ;
#7463=EDGE_LOOP ( 'NONE', ( #6211, #4407, #6224, #11902 ) ) ;
#7464=CARTESIAN_POINT ( 'NONE',  ( -11.52662650599092409, 0.000000000000000000, 3.647599401157420651 ) ) ;
#7465=ADVANCED_FACE ( 'NONE', ( #10259 ), #11606, .F. ) ;
#7472=DIRECTION ( 'NONE',  ( -0.000000000000000000, -1.000000000000000000, -0.000000000000000000 ) ) ;
#7474=CARTESIAN_POINT ( 'NONE',  ( -11.13895890373326836, 0.000000000000000000, 7.723663868796768028 ) ) ;
#7475=CARTESIAN_POINT ( 'NONE',  ( 0.000000000000000000, 3.000000000000000000, 0.000000000000000000 ) ) ;
#7476=CARTESIAN_POINT ( 'NONE',  ( -4.056222772158361245, 0.000000000000000000, 12.16218796965919324 ) ) ;
#7482=AXIS2_PLACEMENT_3D ( 'NONE', #4987, #1826, #5195 ) ;
#7487=CARTESIAN_POINT ( 'NONE',  ( 2.568302020731520141, 0.000000000000000000, 12.56087513340552420 ) ) ;
#7491=CARTESIAN_POINT ( 'NONE',  ( 0.5398653231797245766, 0.000000000000000000, -12.07794044664754018 ) ) ;
#7493=VECTOR ( 'NONE', #199, 1000.000000000000000 ) ;
#7496=CARTESIAN_POINT ( 'NONE',  ( -8.914835885878215294, 3.000000000000000000, 11.11702303352197063 ) ) ;
#7497=ORIENTED_EDGE ( 'NONE', *, *, #4220, .F. ) ;
#7498=CARTESIAN_POINT ( 'NONE',  ( 0.000000000000000000, 0.000000000000000000, 0.000000000000000000 ) ) ;
#7499=PRESENTATION_STYLE_ASSIGNMENT (( #8322 ) ) ;
#7501=EDGE_CURVE ( 'NONE', #6311, #1501, #128, .T. ) ;
#7507=CARTESIAN_POINT ( 'NONE',  ( -4.056222772158361245, 3.000000000000000000, 12.16218796965919324 ) ) ;
#7508=FACE_OUTER_BOUND ( 'NONE', #8677, .T. ) ;
#7512=ORIENTED_EDGE ( 'NONE', *, *, #2615, .F. ) ;
#7518=ORIENTED_EDGE ( 'NONE', *, *, #3970, .F. ) ;
#7519=CARTESIAN_POINT ( 'NONE',  ( -12.07794044664754018, 3.000000000000000000, -0.5398653231797256868 ) ) ;
#7520=LINE ( 'NONE', #4284, #4950 ) ;
#7524=CARTESIAN_POINT ( 'NONE',  ( 0.000000000000000000, 3.000000000000000000, 0.000000000000000000 ) ) ;
#7528=LINE ( 'NONE', #5658, #3615 ) ;
#7530=CARTESIAN_POINT ( 'NONE',  ( -12.14623037080100865, 0.000000000000000000, 4.072642252455982437 ) ) ;
#7532=EDGE_CURVE ( 'NONE', #7218, #12590, #2468, .T. ) ;
#7535=ORIENTED_EDGE ( 'NONE', *, *, #10402, .T. ) ;
#7541=EDGE_CURVE ( 'NONE', #10341, #1734, #3744, .T. ) ;
#7542=CARTESIAN_POINT ( 'NONE',  ( 10.18987059060247269, 0.000000000000000000, 6.506507307819714647 ) ) ;
#7544=DIRECTION ( 'NONE',  ( 0.000000000000000000, 1.000000000000000000, 0.000000000000000000 ) ) ;
#7548=CIRCLE ( 'NONE', #3805, 12.08999999999737440 ) ;
#7550=ORIENTED_EDGE ( 'NONE', *, *, #1183, .F. ) ;
#7559=CARTESIAN_POINT ( 'NONE',  ( -11.52666717836884125, 0.000000000000000000, -3.647470871583627705 ) ) ;
#7563=CARTESIAN_POINT ( 'NONE',  ( 0.000000000000000000, 3.000000000000000000, 0.000000000000000000 ) ) ;
#7564=AXIS2_PLACEMENT_3D ( 'NONE', #6132, #5100, #7112 ) ;
#7565=ORIENTED_EDGE ( 'NONE', *, *, #7752, .T. ) ;
#7566=ORIENTED_EDGE ( 'NONE', *, *, #7272, .F. ) ;
#7567=ORIENTED_EDGE ( 'NONE', *, *, #2961, .T. ) ;
#7579=CARTESIAN_POINT ( 'NONE',  ( 0.000000000000000000, 3.000000000000000000, 0.000000000000000000 ) ) ;
#7580=VERTEX_POINT ( 'NONE', #6369 ) ;
#7597=CARTESIAN_POINT ( 'NONE',  ( -2.161962830978702677, 0.000000000000000000, 14.08504230442587435 ) ) ;
#7599=CARTESIAN_POINT ( 'NONE',  ( 2.604399508763947768, 0.000000000000000000, -11.80615107470197778 ) ) ;
#7604=CARTESIAN_POINT ( 'NONE',  ( 2.161962830978677363, 0.000000000000000000, 14.08504230442587613 ) ) ;
#7607=ADVANCED_FACE ( 'NONE', ( #10849 ), #1275, .T. ) ;
#7609=DIRECTION ( 'NONE',  ( 0.000000000000000000, 0.000000000000000000, 1.000000000000000000 ) ) ;
#7619=ORIENTED_EDGE ( 'NONE', *, *, #6952, .F. ) ;
#7620=CARTESIAN_POINT ( 'NONE',  ( 11.11702303352196708, 0.000000000000000000, 8.914835885878218846 ) ) ;
#7621=EDGE_CURVE ( 'NONE', #2502, #11941, #2441, .T. ) ;
#7627=CARTESIAN_POINT ( 'NONE',  ( -13.04554897075795949, 3.000000000000000000, 5.733772933379550629 ) ) ;
#7628=B_SPLINE_SURFACE_WITH_KNOTS ( 'NONE', 3, 1, ( 
 ( #6316, #12671 ),
 ( #3147, #5353 ),
 ( #959, #3270 ),
 ( #140, #146 ) ),
 .UNSPECIFIED., .F., .F., .F.,
 ( 4, 4 ),
 ( 2, 2 ),
 ( 0.2280192144657617603, 0.8452273900860258760 ),
 ( 0.000000000000000000, 1.000000000000000000 ),
 .UNSPECIFIED. ) ;
#7637=CARTESIAN_POINT ( 'NONE',  ( 1.119409668803368119, 0.000000000000000000, 13.50845331674225847 ) ) ;
#7640=B_SPLINE_SURFACE_WITH_KNOTS ( 'NONE', 3, 1, ( 
 ( #11694, #6590 ),
 ( #2332, #4256 ),
 ( #1357, #9758 ),
 ( #74, #4388 ) ),
 .UNSPECIFIED., .F., .F., .F.,
 ( 4, 4 ),
 ( 2, 2 ),
 ( 0.1547128134717859205, 1.000000000000000000 ),
 ( 0.000000000000000000, 1.000000000000000000 ),
 .UNSPECIFIED. ) ;
#7649=ORIENTED_EDGE ( 'NONE', *, *, #6154, .T. ) ;
#7653=B_SPLINE_CURVE_WITH_KNOTS ( 'NONE', 3,
 ( #11221, #829, #3022, #7230 ),
 .UNSPECIFIED., .F., .F.,
 ( 4, 4 ),
 ( 0.000000000000000000, 0.8452273900860258760 ),
 .UNSPECIFIED. ) ;
#7660=EDGE_CURVE ( 'NONE', #5111, #9128, #8191, .T. ) ;
#7663=ORIENTED_EDGE ( 'NONE', *, *, #10526, .F. ) ;
#7664=ORIENTED_EDGE ( 'NONE', *, *, #11017, .F. ) ;
#7668=CARTESIAN_POINT ( 'NONE',  ( 4.564691384634508964, 0.000000000000000000, -12.76342233970727413 ) ) ;
#7671=EDGE_CURVE ( 'NONE', #11851, #7415, #4228, .T. ) ;
#7673=DIRECTION ( 'NONE',  ( 1.000000000000000000, -0.000000000000000000, -9.145772869372436484E-17 ) ) ;
#7677=EDGE_CURVE ( 'NONE', #8335, #11680, #299, .T. ) ;
#7678=ORIENTED_EDGE ( 'NONE', *, *, #9257, .T. ) ;
#7679=ADVANCED_FACE ( 'NONE', ( #10774 ), #8828, .T. ) ;
#7684=CYLINDRICAL_SURFACE ( 'NONE', #79, 14.25000000000000178 ) ;
#7690=CARTESIAN_POINT ( 'NONE',  ( -5.170206418547117266, 0.000000000000000000, 13.27898586450088203 ) ) ;
#7695=CARTESIAN_POINT ( 'NONE',  ( 0.7901945867173618687, 0.000000000000000000, 12.78643498603817541 ) ) ;
#7698=VERTEX_POINT ( 'NONE', #1417 ) ;
#7699=DIRECTION ( 'NONE',  ( -0.000000000000000000, -1.000000000000000000, -0.000000000000000000 ) ) ;
#7701=CARTESIAN_POINT ( 'NONE',  ( 0.000000000000000000, 3.000000000000000000, 0.000000000000000000 ) ) ;
#7707=FACE_OUTER_BOUND ( 'NONE', #6531, .T. ) ;
#7714=EDGE_LOOP ( 'NONE', ( #11266, #7026, #1109, #1420 ) ) ;
#7721=FACE_OUTER_BOUND ( 'NONE', #1360, .T. ) ;
#7722=CARTESIAN_POINT ( 'NONE',  ( 2.546103534247748712, 3.000000000000000000, -12.55526518755974585 ) ) ;
#7723=CARTESIAN_POINT ( 'NONE',  ( -11.11702303352192445, 3.000000000000000000, 8.914835885878272137 ) ) ;
#7726=DIRECTION ( 'NONE',  ( 0.000000000000000000, 1.000000000000000000, 0.000000000000000000 ) ) ;
#7736=CARTESIAN_POINT ( 'NONE',  ( 11.48836750521728511, 0.000000000000000000, 8.430890348300561499 ) ) ;
#7737=CARTESIAN_POINT ( 'NONE',  ( 2.161962830978694683, 3.000000000000000000, -14.08504230442587790 ) ) ;
#7746=EDGE_CURVE ( 'NONE', #8499, #6668, #12600, .T. ) ;
#7749=FACE_OUTER_BOUND ( 'NONE', #2319, .T. ) ;
#7750=CARTESIAN_POINT ( 'NONE',  ( 6.506620931068708202, 0.000000000000000000, 10.18979803820052155 ) ) ;
#7752=EDGE_CURVE ( 'NONE', #1864, #8421, #484, .T. ) ;
#7761=CARTESIAN_POINT ( 'NONE',  ( 0.000000000000000000, 3.000000000000000000, 0.000000000000000000 ) ) ;
#7768=CARTESIAN_POINT ( 'NONE',  ( -6.506620931068619385, 0.000000000000000000, -10.18979803820057306 ) ) ;
#7770=EDGE_LOOP ( 'NONE', ( #9369, #774, #3394, #9628 ) ) ;
#7773=DIRECTION ( 'NONE',  ( -0.000000000000000000, -1.000000000000000000, -0.000000000000000000 ) ) ;
#7776=AXIS2_PLACEMENT_3D ( 'NONE', #11707, #4342, #5369 ) ;
#7777=CYLINDRICAL_SURFACE ( 'NONE', #10387, 12.08999999999737440 ) ;
#7780=DIRECTION ( 'NONE',  ( 0.000000000000000000, 1.000000000000000000, 0.000000000000000000 ) ) ;
#7786=VERTEX_POINT ( 'NONE', #11127 ) ;
#7787=CIRCLE ( 'NONE', #773, 12.08999999999737440 ) ;
#7791=DIRECTION ( 'NONE',  ( 0.000000000000000000, 1.000000000000000000, 0.000000000000000000 ) ) ;
#7800=ORIENTED_EDGE ( 'NONE', *, *, #1148, .F. ) ;
#7802=CARTESIAN_POINT ( 'NONE',  ( 8.430890348300625448, 0.000000000000000000, 11.48836750521723893 ) ) ;
#7804=CARTESIAN_POINT ( 'NONE',  ( 4.056222772158357692, 0.000000000000000000, -12.16218796965919680 ) ) ;
#7805=CARTESIAN_POINT ( 'NONE',  ( -14.08504230442586369, 3.000000000000000000, 2.161962830978784389 ) ) ;
#7810=CARTESIAN_POINT ( 'NONE',  ( 13.27898586450067242, 3.000000000000000000, -5.170206418547655502 ) ) ;
#7811=EDGE_LOOP ( 'NONE', ( #7990, #2739, #94, #9580 ) ) ;
#7814=EDGE_LOOP ( 'NONE', ( #11938, #8781, #2534, #2680 ) ) ;
#7815=ORIENTED_EDGE ( 'NONE', *, *, #1799, .T. ) ;
#7817=CARTESIAN_POINT ( 'NONE',  ( 0.000000000000000000, 3.000000000000000000, 0.000000000000000000 ) ) ;
#7818=DIRECTION ( 'NONE',  ( 0.000000000000000000, 1.000000000000000000, 0.000000000000000000 ) ) ;
#7821=CARTESIAN_POINT ( 'NONE',  ( 0.000000000000000000, 3.000000000000000000, 0.000000000000000000 ) ) ;
#7823=EDGE_CURVE ( 'NONE', #1734, #10022, #13187, .T. ) ;
#7827=ORIENTED_EDGE ( 'NONE', *, *, #4220, .T. ) ;
#7829=ORIENTED_EDGE ( 'NONE', *, *, #6917, .F. ) ;
#7831=ADVANCED_FACE ( 'NONE', ( #4923 ), #8617, .F. ) ;
#7832=VERTEX_POINT ( 'NONE', #8909 ) ;
#7833=CARTESIAN_POINT ( 'NONE',  ( 5.733772933379474246, 0.000000000000000000, -13.04554897075799502 ) ) ;
#7835=DIRECTION ( 'NONE',  ( 0.000000000000000000, 1.000000000000000000, 0.000000000000000000 ) ) ;
#7840=EDGE_LOOP ( 'NONE', ( #5691, #8739, #709, #6328 ) ) ;
#7841=FACE_OUTER_BOUND ( 'NONE', #6565, .T. ) ;
#7843=EDGE_CURVE ( 'NONE', #5502, #9963, #803, .T. ) ;
#7846=ADVANCED_FACE ( 'NONE', ( #2641 ), #6848, .F. ) ;
#7847=ADVANCED_BREP_SHAPE_REPRESENTATION ( '', ( #8440, #10007 ), #5843 ) ;
#7848=ORIENTED_EDGE ( 'NONE', *, *, #8846, .T. ) ;
#7853=CARTESIAN_POINT ( 'NONE',  ( -13.50845331674225847, 3.000000000000000000, 1.119409668803372115 ) ) ;
#7854=CARTESIAN_POINT ( 'NONE',  ( 8.914835885878220623, 3.000000000000000000, -11.11702303352196708 ) ) ;
#7859=VERTEX_POINT ( 'NONE', #6292 ) ;
#7863=LINE ( 'NONE', #436, #4506 ) ;
#7864=LINE ( 'NONE', #9033, #9295 ) ;
#7865=LINE ( 'NONE', #10145, #4611 ) ;
#7867=B_SPLINE_CURVE_WITH_KNOTS ( 'NONE', 3,
 ( #1530, #10130, #4770, #4901 ),
 .UNSPECIFIED., .F., .F.,
 ( 4, 4 ),
 ( 0.000000000000000000, 0.8452273900860258760 ),
 .UNSPECIFIED. ) ;
#7872=CARTESIAN_POINT ( 'NONE',  ( 12.03251085770905959, 3.000000000000000000, 3.999999998926332179 ) ) ;
#7873=ADVANCED_FACE ( 'NONE', ( #11337 ), #12517, .T. ) ;
#7879=CARTESIAN_POINT ( 'NONE',  ( 1.557181465540672161, 3.000000000000000000, -14.16466328168010591 ) ) ;
#7880=DIRECTION ( 'NONE',  ( -0.000000000000000000, -1.000000000000000000, -0.000000000000000000 ) ) ;
#7885=DIRECTION ( 'NONE',  ( -0.000000000000000000, -1.000000000000000000, -0.000000000000000000 ) ) ;
#7886=LINE ( 'NONE', #3758, #8210 ) ;
#7891=ORIENTED_EDGE ( 'NONE', *, *, #4572, .T. ) ;
#7894=CARTESIAN_POINT ( 'NONE',  ( 10.18987059060247269, 3.000000000000000000, 6.506507307819714647 ) ) ;
#7906=VERTEX_POINT ( 'NONE', #3194 ) ;
#7908=ORIENTED_EDGE ( 'NONE', *, *, #2953, .T. ) ;
#7909=CARTESIAN_POINT ( 'NONE',  ( -7.065816209474154341, 0.000000000000000000, 10.69794375946289833 ) ) ;
#7913=EDGE_CURVE ( 'NONE', #1800, #7218, #7330, .T. ) ;
#7914=DIRECTION ( 'NONE',  ( 0.000000000000000000, 1.000000000000000000, 0.000000000000000000 ) ) ;
#7915=VECTOR ( 'NONE', #12375, 1000.000000000000000 ) ;
#7918=DIRECTION ( 'NONE',  ( 0.000000000000000000, 0.000000000000000000, 1.000000000000000000 ) ) ;
#7921=CARTESIAN_POINT ( 'NONE',  ( -8.430890348300632553, 3.000000000000000000, -11.48836750521723538 ) ) ;
#7924=CARTESIAN_POINT ( 'NONE',  ( -0.5400000000008023937, 3.000000000000000000, -12.07793442604883971 ) ) ;
#7932=EDGE_CURVE ( 'NONE', #9350, #8654, #6361, .T. ) ;
#7934=CARTESIAN_POINT ( 'NONE',  ( -5.571313494980134173, 0.000000000000000000, 10.72979803820131295 ) ) ;
#7935=ADVANCED_FACE ( 'NONE', ( #2098 ), #12809, .F. ) ;
#7941=ADVANCED_FACE ( 'NONE', ( #10295 ), #8290, .F. ) ;
#7942=VECTOR ( 'NONE', #5817, 1000.000000000000000 ) ;
#7952=CARTESIAN_POINT ( 'NONE',  ( 6.506507307819716424, 3.000000000000000000, -10.18987059060247269 ) ) ;
#7953=CARTESIAN_POINT ( 'NONE',  ( 7.077546079049268357, 3.000000000000000000, 10.67828022838850544 ) ) ;
#7959=B_SPLINE_SURFACE_WITH_KNOTS ( 'NONE', 3, 1, ( 
 ( #2545, #8544 ),
 ( #7459, #11659 ),
 ( #1193, #1927 ),
 ( #8049, #7976 ) ),
 .UNSPECIFIED., .F., .F., .F.,
 ( 4, 4 ),
 ( 2, 2 ),
 ( 0.000000000000000000, 0.8452273900860258760 ),
 ( 0.000000000000000000, 1.000000000000000000 ),
 .UNSPECIFIED. ) ;
#7970=VECTOR ( 'NONE', #9236, 1000.000000000000000 ) ;
#7973=CARTESIAN_POINT ( 'NONE',  ( 6.506620931068707314, 3.000000000000000000, 10.18979803820051622 ) ) ;
#7976=CARTESIAN_POINT ( 'NONE',  ( -11.52666717836884125, 0.000000000000000000, -3.647470871583627705 ) ) ;
#7977=DIRECTION ( 'NONE',  ( 0.000000000000000000, 1.000000000000000000, 0.000000000000000000 ) ) ;
#7980=ORIENTED_EDGE ( 'NONE', *, *, #151, .F. ) ;
#7985=EDGE_CURVE ( 'NONE', #9002, #1142, #12457, .T. ) ;
#7990=ORIENTED_EDGE ( 'NONE', *, *, #12040, .T. ) ;
#7997=CARTESIAN_POINT ( 'NONE',  ( -0.5400000000007666445, 0.000000000000000000, -12.07793442604883793 ) ) ;
#7998=CARTESIAN_POINT ( 'NONE',  ( 8.158551673544282679, 3.000000000000000000, -8.922226997226884393 ) ) ;
#8007=ORIENTED_EDGE ( 'NONE', *, *, #3956, .F. ) ;
#8010=CARTESIAN_POINT ( 'NONE',  ( 8.922136023539611216, 3.000000000000000000, -8.158651161643899030 ) ) ;
#8015=CARTESIAN_POINT ( 'NONE',  ( 0.000000000000000000, 3.000000000000000000, 0.000000000000000000 ) ) ;
#8019=CARTESIAN_POINT ( 'NONE',  ( 10.67828022838850366, 0.000000000000000000, -7.077546079049271022 ) ) ;
#8025=AXIS2_PLACEMENT_3D ( 'NONE', #11344, #6040, #11408 ) ;
#8026=CIRCLE ( 'NONE', #13535, 14.25000000000000000 ) ;
#8030=CARTESIAN_POINT ( 'NONE',  ( 0.000000000000000000, 3.000000000000000000, 0.000000000000000000 ) ) ;
#8036=EDGE_CURVE ( 'NONE', #911, #10812, #2916, .T. ) ;
#8038=EDGE_CURVE ( 'NONE', #9443, #7142, #9522, .T. ) ;
#8042=ORIENTED_EDGE ( 'NONE', *, *, #4993, .T. ) ;
#8044=ORIENTED_EDGE ( 'NONE', *, *, #8764, .F. ) ;
#8046=DIRECTION ( 'NONE',  ( -0.000000000000000000, -1.000000000000000000, -0.000000000000000000 ) ) ;
#8048=CARTESIAN_POINT ( 'NONE',  ( -6.506507307819711095, 3.000000000000000000, 10.18987059060247624 ) ) ;
#8049=CARTESIAN_POINT ( 'NONE',  ( -11.52666717836884125, 3.000000000000000000, -3.647470871583627705 ) ) ;
#8051=B_SPLINE_CURVE_WITH_KNOTS ( 'NONE', 3,
 ( #1230, #10789, #8451, #6660 ),
 .UNSPECIFIED., .F., .F.,
 ( 4, 4 ),
 ( 0.000000000000000000, 0.8452273900860258760 ),
 .UNSPECIFIED. ) ;
#8053=EDGE_CURVE ( 'NONE', #7859, #1406, #11285, .T. ) ;
#8058=ORIENTED_EDGE ( 'NONE', *, *, #7823, .F. ) ;
#8060=VERTEX_POINT ( 'NONE', #7604 ) ;
#8064=CARTESIAN_POINT ( 'NONE',  ( 8.158551673544282679, 0.000000000000000000, -8.922226997226884393 ) ) ;
#8067=( LENGTH_UNIT ( ) NAMED_UNIT ( * ) SI_UNIT ( .MILLI., .METRE. ) );
#8069=CARTESIAN_POINT ( 'NONE',  ( -1.557181465540760534, 0.000000000000000000, -14.16466328168009703 ) ) ;
#8071=CARTESIAN_POINT ( 'NONE',  ( 10.72973591378220704, 3.000000000000000000, -5.571433138827823761 ) ) ;
#8074=CARTESIAN_POINT ( 'NONE',  ( -5.708888906988910605, 3.000000000000000000, 11.46847481510586597 ) ) ;
#8085=EDGE_CURVE ( 'NONE', #10517, #5245, #5693, .T. ) ;
#8089=CARTESIAN_POINT ( 'NONE',  ( 10.18979803820052155, 3.000000000000000000, -6.506620931068708202 ) ) ;
#8092=ORIENTED_EDGE ( 'NONE', *, *, #1270, .T. ) ;
#8093=VERTEX_POINT ( 'NONE', #4362 ) ;
#8095=DIRECTION ( 'NONE',  ( 0.000000000000000000, 1.000000000000000000, 0.000000000000000000 ) ) ;
#8101=EDGE_CURVE ( 'NONE', #8964, #5111, #5549, .T. ) ;
#8105=CARTESIAN_POINT ( 'NONE',  ( 10.72973591378220704, 3.000000000000000000, -5.571433138827823761 ) ) ;
#8106=ORIENTED_EDGE ( 'NONE', *, *, #8881, .T. ) ;
#8108=CARTESIAN_POINT ( 'NONE',  ( -11.48836750521728689, 3.000000000000000000, -8.430890348300561499 ) ) ;
#8111=CARTESIAN_POINT ( 'NONE',  ( 9.593885948927676210, 0.000000000000000000, -8.504652361247169168 ) ) ;
#8115=DIRECTION ( 'NONE',  ( 0.000000000000000000, 1.000000000000000000, 0.000000000000000000 ) ) ;
#8118=ORIENTED_EDGE ( 'NONE', *, *, #5555, .T. ) ;
#8124=VERTEX_POINT ( 'NONE', #307 ) ;
#8141=CARTESIAN_POINT ( 'NONE',  ( 8.158651161643900807, 3.000000000000000000, 8.922136023539609440 ) ) ;
#8148=CARTESIAN_POINT ( 'NONE',  ( -1.119409668803374558, 0.000000000000000000, -13.50845331674225669 ) ) ;
#8150=CIRCLE ( 'NONE', #1560, 14.25000000000000000 ) ;
#8153=ORIENTED_EDGE ( 'NONE', *, *, #10021, .F. ) ;
#8162=CARTESIAN_POINT ( 'NONE',  ( 6.506507307819716424, 3.000000000000000000, -10.18987059060247269 ) ) ;
#8168=EDGE_CURVE ( 'NONE', #2208, #3304, #9319, .T. ) ;
#8170=ORIENTED_EDGE ( 'NONE', *, *, #2799, .F. ) ;
#8171=EDGE_CURVE ( 'NONE', #13138, #7859, #12077, .T. ) ;
#8176=AXIS2_PLACEMENT_3D ( 'NONE', #3673, #12241, #4719 ) ;
#8177=CARTESIAN_POINT ( 'NONE',  ( -12.55526518755974585, 0.000000000000000000, -2.546103534247746047 ) ) ;
#8180=CARTESIAN_POINT ( 'NONE',  ( -2.161962830978783057, 3.000000000000000000, -14.08504230442586369 ) ) ;
#8181=CARTESIAN_POINT ( 'NONE',  ( -11.11702303352197063, 3.000000000000000000, -8.914835885878215294 ) ) ;
#8191=B_SPLINE_CURVE_WITH_KNOTS ( 'NONE', 3,
 ( #1215, #12031, #9872, #11878 ),
 .UNSPECIFIED., .F., .F.,
 ( 4, 4 ),
 ( 0.000000000000000000, 0.8452273900860258760 ),
 .UNSPECIFIED. ) ;
#8196=DIRECTION ( 'NONE',  ( 0.000000000000000000, 0.000000000000000000, -1.000000000000000000 ) ) ;
#8199=FACE_OUTER_BOUND ( 'NONE', #8635, .T. ) ;
#8200=ORIENTED_EDGE ( 'NONE', *, *, #8696, .T. ) ;
#8203=ORIENTED_EDGE ( 'NONE', *, *, #6982, .T. ) ;
#8208=VECTOR ( 'NONE', #2775, 1000.000000000000000 ) ;
#8210=VECTOR ( 'NONE', #8779, 1000.000000000000000 ) ;
#8215=CARTESIAN_POINT ( 'NONE',  ( 12.01285915242476499, 3.000000000000000000, -4.000000001073668265 ) ) ;
#8217=CARTESIAN_POINT ( 'NONE',  ( 0.000000000000000000, 0.000000000000000000, 0.000000000000000000 ) ) ;
#8218=CARTESIAN_POINT ( 'NONE',  ( 31.00000000000000000, 3.000000000000000000, -1.500000000759764029 ) ) ;
#8221=CARTESIAN_POINT ( 'NONE',  ( 12.25282671965375592, 3.000000000000000000, -5.797378255456012930 ) ) ;
#8224=ORIENTED_EDGE ( 'NONE', *, *, #8932, .F. ) ;
#8225=ORIENTED_EDGE ( 'NONE', *, *, #10901, .F. ) ;
#8232=CARTESIAN_POINT ( 'NONE',  ( 10.72973591378220704, 0.000000000000000000, -5.571433138827823761 ) ) ;
#8236=CARTESIAN_POINT ( 'NONE',  ( 0.000000000000000000, 0.000000000000000000, 0.000000000000000000 ) ) ;
#8242=CIRCLE ( 'NONE', #11549, 12.08999999999737440 ) ;
#8245=B_SPLINE_CURVE_WITH_KNOTS ( 'NONE', 3,
 ( #1000, #1196, #3833, #7400 ),
 .UNSPECIFIED., .F., .F.,
 ( 4, 4 ),
 ( 0.000000000000000000, 0.8452273900860258760 ),
 .UNSPECIFIED. ) ;
#8252=EDGE_CURVE ( 'NONE', #9891, #1728, #4014, .T. ) ;
#8254=EDGE_CURVE ( 'NONE', #11718, #8926, #8645, .T. ) ;
#8259=STYLED_ITEM ( 'NONE', ( #7499 ), #7847 ) ;
#8281=CARTESIAN_POINT ( 'NONE',  ( 6.506620931068707314, 3.000000000000000000, 10.18979803820051622 ) ) ;
#8282=DIRECTION ( 'NONE',  ( -0.000000000000000000, -1.000000000000000000, -0.000000000000000000 ) ) ;
#8283=CARTESIAN_POINT ( 'NONE',  ( -5.708888906988910605, 3.000000000000000000, 11.46847481510586597 ) ) ;
#8288=B_SPLINE_CURVE_WITH_KNOTS ( 'NONE', 3,
 ( #8281, #8408, #13531, #5116 ),
 .UNSPECIFIED., .F., .F.,
 ( 4, 4 ),
 ( 0.1547128134717859205, 1.000000000000000000 ),
 .UNSPECIFIED. ) ;
#8289=EDGE_LOOP ( 'NONE', ( #1713, #11224, #7369, #1983 ) ) ;
#8290=CYLINDRICAL_SURFACE ( 'NONE', #4238, 1.500000000000000222 ) ;
#8293=ORIENTED_EDGE ( 'NONE', *, *, #2334, .F. ) ;
#8296=CARTESIAN_POINT ( 'NONE',  ( 11.11702303352194043, 3.000000000000000000, -8.914835885878249044 ) ) ;
#8309=DIRECTION ( 'NONE',  ( 0.000000000000000000, 0.000000000000000000, 1.000000000000000000 ) ) ;
#8320=VERTEX_POINT ( 'NONE', #2904 ) ;
#8322=SURFACE_STYLE_USAGE ( .BOTH. , #10680 ) ;
#8329=CARTESIAN_POINT ( 'NONE',  ( -11.11702303352192445, 0.000000000000000000, 8.914835885878272137 ) ) ;
#8335=VERTEX_POINT ( 'NONE', #4975 ) ;
#8337=EDGE_CURVE ( 'NONE', #6519, #6591, #9538, .T. ) ;
#8339=EDGE_CURVE ( 'NONE', #11537, #313, #7548, .T. ) ;
#8341=FACE_OUTER_BOUND ( 'NONE', #12472, .T. ) ;
#8342=AXIS2_PLACEMENT_3D ( 'NONE', #547, #8861, #12885 ) ;
#8346=FACE_OUTER_BOUND ( 'NONE', #6613, .T. ) ;
#8349=EDGE_LOOP ( 'NONE', ( #1730, #4154, #10614, #1947 ) ) ;
#8351=CIRCLE ( 'NONE', #13195, 14.25000000000000178 ) ;
#8355=VERTEX_POINT ( 'NONE', #9439 ) ;
#8356=CARTESIAN_POINT ( 'NONE',  ( -1.557181465540221188, 3.000000000000000000, 14.16466328168015743 ) ) ;
#8359=CIRCLE ( 'NONE', #10126, 14.25000000000000000 ) ;
#8362=CARTESIAN_POINT ( 'NONE',  ( 7.065816209474156118, 0.000000000000000000, -10.69794375946289833 ) ) ;
#8364=B_SPLINE_CURVE_WITH_KNOTS ( 'NONE', 3,
 ( #2601, #5696, #1299, #7894 ),
 .UNSPECIFIED., .F., .F.,
 ( 4, 4 ),
 ( 0.000000000000000000, 0.8452273900860258760 ),
 .UNSPECIFIED. ) ;
#8366=VERTEX_POINT ( 'NONE', #979 ) ;
#8370=AXIS2_PLACEMENT_3D ( 'NONE', #7821, #2249, #3416 ) ;
#8371=ORIENTED_EDGE ( 'NONE', *, *, #9345, .T. ) ;
#8380=DIRECTION ( 'NONE',  ( -0.000000000000000000, -1.000000000000000000, -0.000000000000000000 ) ) ;
#8384=VERTEX_POINT ( 'NONE', #8329 ) ;
#8394=EDGE_CURVE ( 'NONE', #11839, #2012, #1175, .T. ) ;
#8400=ORIENTED_EDGE ( 'NONE', *, *, #9345, .F. ) ;
#8404=AXIS2_PLACEMENT_3D ( 'NONE', #99, #7452, #164 ) ;
#8406=AXIS2_PLACEMENT_3D ( 'NONE', #1805, #3031, #11434 ) ;
#8408=CARTESIAN_POINT ( 'NONE',  ( 7.077546079049268357, 3.000000000000000000, 10.67828022838850544 ) ) ;
#8414=CARTESIAN_POINT ( 'NONE',  ( -6.506620931068619385, 3.000000000000000000, -10.18979803820057306 ) ) ;
#8417=ORIENTED_EDGE ( 'NONE', *, *, #1455, .F. ) ;
#8418=CARTESIAN_POINT ( 'NONE',  ( 4.577511697546072789, 0.000000000000000000, 12.75843939030335505 ) ) ;
#8419=ORIENTED_EDGE ( 'NONE', *, *, #11688, .T. ) ;
#8421=VERTEX_POINT ( 'NONE', #4000 ) ;
#8424=ORIENTED_EDGE ( 'NONE', *, *, #4323, .F. ) ;
#8430=VECTOR ( 'NONE', #1158, 1000.000000000000000 ) ;
#8436=EDGE_CURVE ( 'NONE', #4189, #6233, #1307, .T. ) ;
#8437=CARTESIAN_POINT ( 'NONE',  ( 10.34346111134700585, 0.000000000000000000, 8.760376775873716326 ) ) ;
#8438=AXIS2_PLACEMENT_3D ( 'NONE', #4592, #8777, #5836 ) ;
#8440=MANIFOLD_SOLID_BREP ( 'Boss-Extrude1', #12598 ) ;
#8444=CYLINDRICAL_SURFACE ( 'NONE', #6147, 1.499999999686092877 ) ;
#8451=CARTESIAN_POINT ( 'NONE',  ( -5.731782959214987372, 3.000000000000000000, -11.46814821560793618 ) ) ;
#8455=ORIENTED_EDGE ( 'NONE', *, *, #11230, .F. ) ;
#8456=VERTEX_POINT ( 'NONE', #1246 ) ;
#8462=DIRECTION ( 'NONE',  ( -0.000000000000000000, -1.000000000000000000, -0.000000000000000000 ) ) ;
#8468=DIRECTION ( 'NONE',  ( 0.000000000000000000, 1.000000000000000000, 0.000000000000000000 ) ) ;
#8473=EDGE_LOOP ( 'NONE', ( #5728, #11029, #9913, #11091 ) ) ;
#8475=CARTESIAN_POINT ( 'NONE',  ( -8.504652361247167391, 0.000000000000000000, -9.593885948927674434 ) ) ;
#8482=FACE_OUTER_BOUND ( 'NONE', #1699, .T. ) ;
#8483=DIRECTION ( 'NONE',  ( 0.000000000000000000, 1.000000000000000000, 0.000000000000000000 ) ) ;
#8484=CARTESIAN_POINT ( 'NONE',  ( -10.72973591378220348, 0.000000000000000000, 5.571433138827830867 ) ) ;
#8485=CARTESIAN_POINT ( 'NONE',  ( -2.604531154829235362, 0.000000000000000000, -11.80612203322752585 ) ) ;
#8487=DIRECTION ( 'NONE',  ( -0.000000000000000000, -1.000000000000000000, -0.000000000000000000 ) ) ;
#8491=EDGE_CURVE ( 'NONE', #4274, #4058, #10747, .T. ) ;
#8494=FACE_OUTER_BOUND ( 'NONE', #5205, .T. ) ;
#8499=VERTEX_POINT ( 'NONE', #8735 ) ;
#8502=B_SPLINE_SURFACE_WITH_KNOTS ( 'NONE', 3, 1, ( 
 ( #4634, #4571 ),
 ( #13177, #7668 ),
 ( #3600, #7804 ),
 ( #5604, #5733 ) ),
 .UNSPECIFIED., .F., .F., .F.,
 ( 4, 4 ),
 ( 2, 2 ),
 ( 0.000000000000000000, 0.8452273900860258760 ),
 ( 0.000000000000000000, 1.000000000000000000 ),
 .UNSPECIFIED. ) ;
#8503=EDGE_CURVE ( 'NONE', #11589, #1091, #13054, .T. ) ;
#8504=EDGE_CURVE ( 'NONE', #11304, #9891, #931, .T. ) ;
#8518=CARTESIAN_POINT ( 'NONE',  ( 0.000000000000000000, 0.000000000000000000, 0.000000000000000000 ) ) ;
#8519=ADVANCED_FACE ( 'NONE', ( #9706 ), #6479, .T. ) ;
#8522=B_SPLINE_CURVE_WITH_KNOTS ( 'NONE', 3,
 ( #8414, #3051, #5197, #3114 ),
 .UNSPECIFIED., .F., .F.,
 ( 4, 4 ),
 ( 0.1547128134717859205, 1.000000000000000000 ),
 .UNSPECIFIED. ) ;
#8527=DIRECTION ( 'NONE',  ( 0.000000000000000000, 0.000000000000000000, -1.000000000000000000 ) ) ;
#8530=ORIENTED_EDGE ( 'NONE', *, *, #11417, .T. ) ;
#8533=ORIENTED_EDGE ( 'NONE', *, *, #11230, .T. ) ;
#8535=CARTESIAN_POINT ( 'NONE',  ( -0.5400000000007666445, 3.000000000000000000, -12.07793442604883793 ) ) ;
#8538=ORIENTED_EDGE ( 'NONE', *, *, #5163, .F. ) ;
#8544=CARTESIAN_POINT ( 'NONE',  ( -13.27898586450070084, 0.000000000000000000, -5.170206418547585336 ) ) ;
#8547=CARTESIAN_POINT ( 'NONE',  ( -13.27898586450066709, 3.000000000000000000, 5.170206418547661720 ) ) ;
#8550=ORIENTED_EDGE ( 'NONE', *, *, #11417, .F. ) ;
#8552=B_SPLINE_CURVE_WITH_KNOTS ( 'NONE', 3,
 ( #7168, #5089, #7229, #10529 ),
 .UNSPECIFIED., .F., .F.,
 ( 4, 4 ),
 ( 0.1547128134717859205, 1.000000000000000000 ),
 .UNSPECIFIED. ) ;
#8553=ORIENTED_EDGE ( 'NONE', *, *, #5916, .T. ) ;
#8556=CARTESIAN_POINT ( 'NONE',  ( -1.105736515254454044, 0.000000000000000000, 13.50994833511691340 ) ) ;
#8559=CARTESIAN_POINT ( 'NONE',  ( 1.105736515254441388, 3.000000000000000000, -13.50994833511691695 ) ) ;
#8560=DIRECTION ( 'NONE',  ( 0.000000000000000000, 0.000000000000000000, 1.000000000000000000 ) ) ;
#8562=CIRCLE ( 'NONE', #9264, 14.25000000000000000 ) ;
#8563=ORIENTED_EDGE ( 'NONE', *, *, #6212, .F. ) ;
#8569=CARTESIAN_POINT ( 'NONE',  ( -9.593885948927676210, 0.000000000000000000, 8.504652361247165615 ) ) ;
#8570=CIRCLE ( 'NONE', #12563, 12.08999999999737263 ) ;
#8571=CARTESIAN_POINT ( 'NONE',  ( 10.72979803820131472, 3.000000000000000000, 5.571313494980131509 ) ) ;
#8572=CARTESIAN_POINT ( 'NONE',  ( 5.571433138827823761, 3.000000000000000000, 10.72973591378220704 ) ) ;
#8573=CARTESIAN_POINT ( 'NONE',  ( -12.76342233970728124, 0.000000000000000000, -4.564691384634500970 ) ) ;
#8582=ADVANCED_FACE ( 'NONE', ( #7841 ), #9839, .T. ) ;
#8583=ORIENTED_EDGE ( 'NONE', *, *, #6244, .T. ) ;
#8589=CYLINDRICAL_SURFACE ( 'NONE', #11891, 1.500000000000000222 ) ;
#8597=ORIENTED_EDGE ( 'NONE', *, *, #4776, .F. ) ;
#8601=ADVANCED_FACE ( 'NONE', ( #10112 ), #2367, .F. ) ;
#8613=EDGE_CURVE ( 'NONE', #1800, #7580, #9080, .T. ) ;
#8614=CARTESIAN_POINT ( 'NONE',  ( 8.158651161643900807, 3.000000000000000000, 8.922136023539609440 ) ) ;
#8615=ORIENTED_EDGE ( 'NONE', *, *, #1274, .T. ) ;
#8617=B_SPLINE_SURFACE_WITH_KNOTS ( 'NONE', 3, 1, ( 
 ( #654, #8974 ),
 ( #2850, #4849 ),
 ( #11261, #9125 ),
 ( #9939, #9044 ) ),
 .UNSPECIFIED., .F., .F., .F.,
 ( 4, 4 ),
 ( 2, 2 ),
 ( 0.1547128134717859205, 1.000000000000000000 ),
 ( 0.000000000000000000, 1.000000000000000000 ),
 .UNSPECIFIED. ) ;
#8620=ORIENTED_EDGE ( 'NONE', *, *, #9452, .T. ) ;
#8628=DIRECTION ( 'NONE',  ( 0.000000000000000000, 0.000000000000000000, 1.000000000000000000 ) ) ;
#8633=( GEOMETRIC_REPRESENTATION_CONTEXT ( 3 ) GLOBAL_UNCERTAINTY_ASSIGNED_CONTEXT ( ( #7233 ) ) GLOBAL_UNIT_ASSIGNED_CONTEXT ( ( #12750, #6547, #2205 ) ) REPRESENTATION_CONTEXT ( 'NONE', 'WORKASPACE' ) );
#8634=ORIENTED_EDGE ( 'NONE', *, *, #61, .F. ) ;
#8635=EDGE_LOOP ( 'NONE', ( #1065, #8837, #6051, #5180 ) ) ;
#8636=CARTESIAN_POINT ( 'NONE',  ( 8.922226997226887946, 3.000000000000000000, 8.158551673544288008 ) ) ;
#8643=EDGE_CURVE ( 'NONE', #11321, #8320, #13246, .T. ) ;
#8645=B_SPLINE_CURVE_WITH_KNOTS ( 'NONE', 3,
 ( #13108, #9998, #13318, #9923 ),
 .UNSPECIFIED., .F., .F.,
 ( 4, 4 ),
 ( 0.1547128134717859205, 1.000000000000000000 ),
 .UNSPECIFIED. ) ;
#8647=CARTESIAN_POINT ( 'NONE',  ( -10.72973591378220348, 3.000000000000000000, 5.571433138827830867 ) ) ;
#8648=CARTESIAN_POINT ( 'NONE',  ( -10.72979803820123479, 3.000000000000000000, -5.571313494980285164 ) ) ;
#8653=EDGE_LOOP ( 'NONE', ( #4352, #8293, #7367, #7815 ) ) ;
#8654=VERTEX_POINT ( 'NONE', #2552 ) ;
#8656=CARTESIAN_POINT ( 'NONE',  ( -8.482622935103766082, 3.000000000000000000, 9.600126836553263487 ) ) ;
#8669=CARTESIAN_POINT ( 'NONE',  ( 0.000000000000000000, 3.000000000000000000, 0.000000000000000000 ) ) ;
#8671=ORIENTED_EDGE ( 'NONE', *, *, #8829, .T. ) ;
#8677=EDGE_LOOP ( 'NONE', ( #6814, #12768, #5888, #10553 ) ) ;
#8683=B_SPLINE_CURVE_WITH_KNOTS ( 'NONE', 3,
 ( #10426, #13593, #13333, #4148 ),
 .UNSPECIFIED., .F., .F.,
 ( 4, 4 ),
 ( 0.1547128134717859205, 1.000000000000000000 ),
 .UNSPECIFIED. ) ;
#8684=EDGE_CURVE ( 'NONE', #10793, #7310, #1028, .T. ) ;
#8687=EDGE_CURVE ( 'NONE', #1063, #500, #7653, .T. ) ;
#8694=ORIENTED_EDGE ( 'NONE', *, *, #7843, .T. ) ;
#8696=EDGE_CURVE ( 'NONE', #11680, #781, #2504, .T. ) ;
#8708=EDGE_CURVE ( 'NONE', #11432, #97, #8963, .T. ) ;
#8712=CARTESIAN_POINT ( 'NONE',  ( 7.077546079049268357, 0.000000000000000000, 10.67828022838850544 ) ) ;
#8713=CARTESIAN_POINT ( 'NONE',  ( -12.75843939030334795, 0.000000000000000000, 4.577511697546079006 ) ) ;
#8721=ORIENTED_EDGE ( 'NONE', *, *, #6435, .T. ) ;
#8724=B_SPLINE_CURVE_WITH_KNOTS ( 'NONE', 3,
 ( #6956, #13013, #6741, #5638 ),
 .UNSPECIFIED., .F., .F.,
 ( 4, 4 ),
 ( 0.1547128134717859205, 1.000000000000000000 ),
 .UNSPECIFIED. ) ;
#8725=ORIENTED_EDGE ( 'NONE', *, *, #3694, .F. ) ;
#8728=B_SPLINE_SURFACE_WITH_KNOTS ( 'NONE', 3, 1, ( 
 ( #2589, #12615 ),
 ( #12687, #3164 ),
 ( #7378, #8713 ),
 ( #3229, #11582 ) ),
 .UNSPECIFIED., .F., .F., .F.,
 ( 4, 4 ),
 ( 2, 2 ),
 ( 0.1547128134717859205, 1.000000000000000000 ),
 ( 0.000000000000000000, 1.000000000000000000 ),
 .UNSPECIFIED. ) ;
#8731=B_SPLINE_CURVE_WITH_KNOTS ( 'NONE', 3,
 ( #5622, #393, #1492, #9199 ),
 .UNSPECIFIED., .F., .F.,
 ( 4, 4 ),
 ( 0.1547128134717859205, 1.000000000000000000 ),
 .UNSPECIFIED. ) ;
#8732=DIRECTION ( 'NONE',  ( 0.000000000000000000, 0.000000000000000000, -1.000000000000000000 ) ) ;
#8735=CARTESIAN_POINT ( 'NONE',  ( -10.72973591378220348, 3.000000000000000000, 5.571433138827830867 ) ) ;
#8738=ADVANCED_FACE ( 'NONE', ( #13369 ), #3676, .F. ) ;
#8739=ORIENTED_EDGE ( 'NONE', *, *, #6648, .F. ) ;
#8743=DIRECTION ( 'NONE',  ( 0.000000000000000000, 1.000000000000000000, 0.000000000000000000 ) ) ;
#8744=CARTESIAN_POINT ( 'NONE',  ( 2.161962830978677363, 3.000000000000000000, 14.08504230442587613 ) ) ;
#8750=DIRECTION ( 'NONE',  ( 0.000000000000000000, 0.000000000000000000, 1.000000000000000000 ) ) ;
#8754=VERTEX_POINT ( 'NONE', #12417 ) ;
#8759=CARTESIAN_POINT ( 'NONE',  ( 11.48836750521728511, 3.000000000000000000, 8.430890348300561499 ) ) ;
#8764=EDGE_CURVE ( 'NONE', #13244, #12420, #4704, .T. ) ;
#8769=EDGE_CURVE ( 'NONE', #11851, #2083, #2126, .T. ) ;
#8771=CARTESIAN_POINT ( 'NONE',  ( -6.506620931068619385, 3.000000000000000000, -10.18979803820057306 ) ) ;
#8772=FACE_OUTER_BOUND ( 'NONE', #9648, .T. ) ;
#8777=DIRECTION ( 'NONE',  ( 0.000000000000000000, 1.000000000000000000, 0.000000000000000000 ) ) ;
#8778=ADVANCED_FACE ( 'NONE', ( #5422 ), #7640, .F. ) ;
#8779=DIRECTION ( 'NONE',  ( -0.000000000000000000, -1.000000000000000000, -0.000000000000000000 ) ) ;
#8780=ORIENTED_EDGE ( 'NONE', *, *, #13446, .F. ) ;
#8781=ORIENTED_EDGE ( 'NONE', *, *, #4492, .F. ) ;
#8784=CARTESIAN_POINT ( 'NONE',  ( -2.568302020731516588, 3.000000000000000000, -12.56087513340552242 ) ) ;
#8786=AXIS2_PLACEMENT_3D ( 'NONE', #11624, #7223, #6247 ) ;
#8789=LINE ( 'NONE', #10388, #453 ) ;
#8793=CIRCLE ( 'NONE', #2643, 14.25000000000000000 ) ;
#8810=ORIENTED_EDGE ( 'NONE', *, *, #1541, .F. ) ;
#8811=B_SPLINE_CURVE_WITH_KNOTS ( 'NONE', 3,
 ( #5367, #152, #6541, #9575 ),
 .UNSPECIFIED., .F., .F.,
 ( 4, 4 ),
 ( 0.000000000000000000, 0.8452273900860258760 ),
 .UNSPECIFIED. ) ;
#8818=CARTESIAN_POINT ( 'NONE',  ( -0.5398653231797316820, 3.000000000000000000, 12.07794044664754018 ) ) ;
#8821=CARTESIAN_POINT ( 'NONE',  ( -12.07794044664754018, 0.000000000000000000, -0.5398653231797256868 ) ) ;
#8827=CARTESIAN_POINT ( 'NONE',  ( 12.01285915242476499, 0.000000000000000000, -4.000000001073668265 ) ) ;
#8828=CYLINDRICAL_SURFACE ( 'NONE', #6860, 14.25000000000000178 ) ;
#8829=EDGE_CURVE ( 'NONE', #11807, #544, #4925, .T. ) ;
#8835=B_SPLINE_SURFACE_WITH_KNOTS ( 'NONE', 3, 1, ( 
 ( #8759, #7736 ),
 ( #12975, #4369 ),
 ( #9868, #11950 ),
 ( #2510, #7542 ) ),
 .UNSPECIFIED., .F., .F., .F.,
 ( 4, 4 ),
 ( 2, 2 ),
 ( 0.000000000000000000, 0.8452273900860258760 ),
 ( 0.000000000000000000, 1.000000000000000000 ),
 .UNSPECIFIED. ) ;
#8837=ORIENTED_EDGE ( 'NONE', *, *, #10197, .F. ) ;
#8838=CARTESIAN_POINT ( 'NONE',  ( -10.72979803820123479, 0.000000000000000000, -5.571313494980285164 ) ) ;
#8840=EDGE_CURVE ( 'NONE', #688, #8093, #6033, .T. ) ;
#8846=EDGE_CURVE ( 'NONE', #13326, #2083, #1089, .T. ) ;
#8852=ORIENTED_EDGE ( 'NONE', *, *, #6982, .F. ) ;
#8853=ORIENTED_EDGE ( 'NONE', *, *, #11788, .T. ) ;
#8855=ORIENTED_EDGE ( 'NONE', *, *, #10486, .F. ) ;
#8861=DIRECTION ( 'NONE',  ( 0.000000000000000000, 1.000000000000000000, 0.000000000000000000 ) ) ;
#8863=PLANE ( 'NONE',  #11448 ) ;
#8867=VECTOR ( 'NONE', #1396, 1000.000000000000000 ) ;
#8870=CARTESIAN_POINT ( 'NONE',  ( 0.5398653231797245766, 0.000000000000000000, -12.07794044664754018 ) ) ;
#8881=EDGE_CURVE ( 'NONE', #6616, #11941, #5851, .T. ) ;
#8886=DIRECTION ( 'NONE',  ( -0.000000000000000000, -1.000000000000000000, -0.000000000000000000 ) ) ;
#8888=DIRECTION ( 'NONE',  ( 0.000000000000000000, 0.000000000000000000, -1.000000000000000000 ) ) ;
#8889=CARTESIAN_POINT ( 'NONE',  ( -1.119409668803374558, 3.000000000000000000, -13.50845331674225669 ) ) ;
#8891=AXIS2_PLACEMENT_3D ( 'NONE', #1331, #2632, #5805 ) ;
#8892=DIRECTION ( 'NONE',  ( -0.000000000000000000, -1.000000000000000000, -0.000000000000000000 ) ) ;
#8895=VECTOR ( 'NONE', #10221, 1000.000000000000000 ) ;
#8898=B_SPLINE_CURVE_WITH_KNOTS ( 'NONE', 3,
 ( #9454, #5255, #13538, #110 ),
 .UNSPECIFIED., .F., .F.,
 ( 4, 4 ),
 ( 0.1547128134717859205, 1.000000000000000000 ),
 .UNSPECIFIED. ) ;
#8901=CARTESIAN_POINT ( 'NONE',  ( -5.733772933379472470, 0.000000000000000000, 13.04554897075799502 ) ) ;
#8903=DIRECTION ( 'NONE',  ( -0.000000000000000000, -1.000000000000000000, -0.000000000000000000 ) ) ;
#8904=CARTESIAN_POINT ( 'NONE',  ( 0.000000000000000000, 0.000000000000000000, 0.000000000000000000 ) ) ;
#8905=LINE ( 'NONE', #6842, #12845 ) ;
#8909=CARTESIAN_POINT ( 'NONE',  ( -3.647599401157625376, 3.000000000000000000, -11.52662650599085836 ) ) ;
#8911=EDGE_LOOP ( 'NONE', ( #11753, #8058, #11900, #11306 ) ) ;
#8912=EDGE_CURVE ( 'NONE', #8499, #11537, #7886, .T. ) ;
#8921=CARTESIAN_POINT ( 'NONE',  ( 12.46219022525837694, 0.000000000000000000, -4.344528055836598845 ) ) ;
#8924=VERTEX_POINT ( 'NONE', #5687 ) ;
#8926=VERTEX_POINT ( 'NONE', #4661 ) ;
#8927=ORIENTED_EDGE ( 'NONE', *, *, #6042, .T. ) ;
#8932=EDGE_CURVE ( 'NONE', #2502, #4277, #9968, .T. ) ;
#8941=ORIENTED_EDGE ( 'NONE', *, *, #3282, .T. ) ;
#8946=CARTESIAN_POINT ( 'NONE',  ( -8.430890348300559722, 0.000000000000000000, 11.48836750521728689 ) ) ;
#8949=VERTEX_POINT ( 'NONE', #1644 ) ;
#8958=PRODUCT ( 'gear-link-1', 'gear-link-1', '', ( #884 ) ) ;
#8963=B_SPLINE_CURVE_WITH_KNOTS ( 'NONE', 3,
 ( #7169, #5224, #3915, #963 ),
 .UNSPECIFIED., .F., .F.,
 ( 4, 4 ),
 ( 0.2280192144657617603, 0.8452273900860258760 ),
 .UNSPECIFIED. ) ;
#8964=VERTEX_POINT ( 'NONE', #13483 ) ;
#8968=CARTESIAN_POINT ( 'NONE',  ( -12.25282671965375236, 0.000000000000000000, 5.797378255456025364 ) ) ;
#8974=CARTESIAN_POINT ( 'NONE',  ( -3.647599401157691545, 0.000000000000000000, -11.52662650599084238 ) ) ;
#8977=ORIENTED_EDGE ( 'NONE', *, *, #11223, .T. ) ;
#8978=CARTESIAN_POINT ( 'NONE',  ( 10.72973591378220704, 0.000000000000000000, -5.571433138827823761 ) ) ;
#8980=CARTESIAN_POINT ( 'NONE',  ( -5.571313494980134173, 3.000000000000000000, 10.72979803820131295 ) ) ;
#8981=DIRECTION ( 'NONE',  ( 0.000000000000000000, 0.000000000000000000, 1.000000000000000000 ) ) ;
#8982=CARTESIAN_POINT ( 'NONE',  ( -11.80612203322752585, 3.000000000000000000, 2.604531154829235362 ) ) ;
#8984=CARTESIAN_POINT ( 'NONE',  ( 0.000000000000000000, 3.000000000000000000, 0.000000000000000000 ) ) ;
#8986=CARTESIAN_POINT ( 'NONE',  ( 12.89546620003432764, 0.000000000000000000, -4.733530556166651415 ) ) ;
#8989=ORIENTED_EDGE ( 'NONE', *, *, #13420, .T. ) ;
#8993=CARTESIAN_POINT ( 'NONE',  ( 10.33484986938308481, 0.000000000000000000, -8.771102293099065861 ) ) ;
#8996=CARTESIAN_POINT ( 'NONE',  ( 1.836970198721030181E-16, 3.000000000000000000, 1.500000000000000222 ) ) ;
#8998=EDGE_CURVE ( 'NONE', #12420, #911, #3821, .T. ) ;
#8999=FACE_BOUND ( 'NONE', #119, .T. ) ;
#9002=VERTEX_POINT ( 'NONE', #5144 ) ;
#9005=VECTOR ( 'NONE', #4716, 1000.000000000000000 ) ;
#9011=CARTESIAN_POINT ( 'NONE',  ( 0.000000000000000000, 3.000000000000000000, 0.000000000000000000 ) ) ;
#9013=CARTESIAN_POINT ( 'NONE',  ( -10.69794375946289655, 0.000000000000000000, -7.065816209474156118 ) ) ;
#9016=EDGE_CURVE ( 'NONE', #4277, #1864, #4022, .T. ) ;
#9017=CARTESIAN_POINT ( 'NONE',  ( 1.119409668803368119, 3.000000000000000000, 13.50845331674225847 ) ) ;
#9018=VECTOR ( 'NONE', #3862, 1000.000000000000000 ) ;
#9022=CARTESIAN_POINT ( 'NONE',  ( 1.557181465540758758, 0.000000000000000000, 14.16466328168009881 ) ) ;
#9025=ADVANCED_FACE ( 'NONE', ( #13414 ), #2241, .F. ) ;
#9026=ORIENTED_EDGE ( 'NONE', *, *, #8171, .F. ) ;
#9029=AXIS2_PLACEMENT_3D ( 'NONE', #5684, #11894, #4590 ) ;
#9033=CARTESIAN_POINT ( 'NONE',  ( -10.18979803820068675, 3.000000000000000000, 6.506620931068438196 ) ) ;
#9040=VECTOR ( 'NONE', #7058, 1000.000000000000000 ) ;
#9041=DIRECTION ( 'NONE',  ( 0.000000000000000000, 0.000000000000000000, 1.000000000000000000 ) ) ;
#9042=LINE ( 'NONE', #652, #7942 ) ;
#9044=CARTESIAN_POINT ( 'NONE',  ( -5.170206418547658167, 0.000000000000000000, -13.27898586450066887 ) ) ;
#9046=VERTEX_POINT ( 'NONE', #13354 ) ;
#9049=CARTESIAN_POINT ( 'NONE',  ( 10.72973591378220704, 3.000000000000000000, -5.571433138827823761 ) ) ;
#9051=FACE_OUTER_BOUND ( 'NONE', #2836, .T. ) ;
#9052=B_SPLINE_CURVE_WITH_KNOTS ( 'NONE', 3,
 ( #5567, #1101, #3231, #2342 ),
 .UNSPECIFIED., .F., .F.,
 ( 4, 4 ),
 ( 0.1547128134717859205, 1.000000000000000000 ),
 .UNSPECIFIED. ) ;
#9064=LINE ( 'NONE', #8108, #5338 ) ;
#9067=AXIS2_PLACEMENT_3D ( 'NONE', #7236, #3088, #4062 ) ;
#9071=CARTESIAN_POINT ( 'NONE',  ( 0.000000000000000000, 0.000000000000000000, 0.000000000000000000 ) ) ;
#9078=DIRECTION ( 'NONE',  ( 0.000000000000000000, 0.000000000000000000, 1.000000000000000000 ) ) ;
#9079=VECTOR ( 'NONE', #13548, 1000.000000000000000 ) ;
#9080=CIRCLE ( 'NONE', #6671, 12.08999999999737440 ) ;
#9081=ORIENTED_EDGE ( 'NONE', *, *, #1207, .T. ) ;
#9082=AXIS2_PLACEMENT_3D ( 'NONE', #1525, #7914, #10957 ) ;
#9085=ADVANCED_FACE ( 'NONE', ( #9270 ), #3337, .F. ) ;
#9092=VECTOR ( 'NONE', #5450, 1000.000000000000000 ) ;
#9112=CARTESIAN_POINT ( 'NONE',  ( -14.08504230442587790, 3.000000000000000000, -2.161962830978695571 ) ) ;
#9115=CARTESIAN_POINT ( 'NONE',  ( -11.46814821560793440, 0.000000000000000000, 5.731782959214994477 ) ) ;
#9124=FACE_OUTER_BOUND ( 'NONE', #10396, .T. ) ;
#9125=CARTESIAN_POINT ( 'NONE',  ( -4.577511697546077230, 0.000000000000000000, -12.75843939030334795 ) ) ;
#9126=ORIENTED_EDGE ( 'NONE', *, *, #3703, .F. ) ;
#9128=VERTEX_POINT ( 'NONE', #8821 ) ;
#9139=CARTESIAN_POINT ( 'NONE',  ( -12.07794044664754018, 3.000000000000000000, -0.5398653231797256868 ) ) ;
#9143=CYLINDRICAL_SURFACE ( 'NONE', #12807, 12.08999999999737440 ) ;
#9144=EDGE_CURVE ( 'NONE', #6668, #313, #7864, .T. ) ;
#9145=DIRECTION ( 'NONE',  ( -0.000000000000000000, -1.000000000000000000, -0.000000000000000000 ) ) ;
#9150=DIRECTION ( 'NONE',  ( -0.000000000000000000, -1.000000000000000000, -0.000000000000000000 ) ) ;
#9153=CARTESIAN_POINT ( 'NONE',  ( 8.914835885878220623, 0.000000000000000000, -11.11702303352196708 ) ) ;
#9162=ORIENTED_EDGE ( 'NONE', *, *, #12173, .T. ) ;
#9163=LINE ( 'NONE', #1737, #4373 ) ;
#9171=DIRECTION ( 'NONE',  ( 0.000000000000000000, 0.000000000000000000, 1.000000000000000000 ) ) ;
#9173=ORIENTED_EDGE ( 'NONE', *, *, #4313, .F. ) ;
#9177=FACE_OUTER_BOUND ( 'NONE', #12202, .T. ) ;
#9182=CARTESIAN_POINT ( 'NONE',  ( -13.27898586450066709, 0.000000000000000000, 5.170206418547661720 ) ) ;
#9185=CARTESIAN_POINT ( 'NONE',  ( -11.11702303352192445, 3.000000000000000000, 8.914835885878272137 ) ) ;
#9187=ORIENTED_EDGE ( 'NONE', *, *, #7913, .T. ) ;
#9192=ORIENTED_EDGE ( 'NONE', *, *, #6435, .F. ) ;
#9193=B_SPLINE_CURVE_WITH_KNOTS ( 'NONE', 3,
 ( #2848, #6027, #4641, #12030 ),
 .UNSPECIFIED., .F., .F.,
 ( 4, 4 ),
 ( 0.000000000000000000, 0.8452273900860258760 ),
 .UNSPECIFIED. ) ;
#9199=CARTESIAN_POINT ( 'NONE',  ( -14.16466328168009881, 0.000000000000000000, 1.557181465540760534 ) ) ;
#9203=VERTEX_POINT ( 'NONE', #13178 ) ;
#9204=ADVANCED_FACE ( 'NONE', ( #6020 ), #9947, .F. ) ;
#9206=CARTESIAN_POINT ( 'NONE',  ( 12.25836857253663581, 3.000000000000000000, 5.784789447945493990 ) ) ;
#9210=CYLINDRICAL_SURFACE ( 'NONE', #6397, 14.25000000000000178 ) ;
#9212=EDGE_CURVE ( 'NONE', #9002, #8355, #12599, .T. ) ;
#9213=CARTESIAN_POINT ( 'NONE',  ( -14.16466328168010769, 3.000000000000000000, -1.557181465540673271 ) ) ;
#9214=CARTESIAN_POINT ( 'NONE',  ( -8.158651161643904359, 3.000000000000000000, -8.922136023539605887 ) ) ;
#9229=DIRECTION ( 'NONE',  ( 0.000000000000000000, 1.000000000000000000, 0.000000000000000000 ) ) ;
#9234=EDGE_LOOP ( 'NONE', ( #342, #7368, #4688, #11518 ) ) ;
#9236=DIRECTION ( 'NONE',  ( -0.000000000000000000, -1.000000000000000000, -0.000000000000000000 ) ) ;
#9243=CARTESIAN_POINT ( 'NONE',  ( -11.80612203322752585, 0.000000000000000000, 2.604531154829235362 ) ) ;
#9244=LINE ( 'NONE', #13532, #4176 ) ;
#9246=DIRECTION ( 'NONE',  ( 0.000000000000000000, 0.000000000000000000, 1.000000000000000000 ) ) ;
#9253=ORIENTED_EDGE ( 'NONE', *, *, #6920, .F. ) ;
#9254=B_SPLINE_CURVE_WITH_KNOTS ( 'NONE', 3,
 ( #3545, #10925, #1562, #2452 ),
 .UNSPECIFIED., .F., .F.,
 ( 4, 4 ),
 ( 0.1547128134717859205, 1.000000000000000000 ),
 .UNSPECIFIED. ) ;
#9257=EDGE_CURVE ( 'NONE', #3224, #10361, #8288, .T. ) ;
#9259=ORIENTED_EDGE ( 'NONE', *, *, #6812, .T. ) ;
#9264=AXIS2_PLACEMENT_3D ( 'NONE', #4105, #1213, #6169 ) ;
#9267=DIRECTION ( 'NONE',  ( 0.000000000000000000, 0.000000000000000000, 1.000000000000000000 ) ) ;
#9268=CARTESIAN_POINT ( 'NONE',  ( 8.430890348300565051, 0.000000000000000000, -11.48836750521728334 ) ) ;
#9270=FACE_OUTER_BOUND ( 'NONE', #8911, .T. ) ;
#9276=VERTEX_POINT ( 'NONE', #1896 ) ;
#9286=CARTESIAN_POINT ( 'NONE',  ( -9.593885948927676210, 0.000000000000000000, 8.504652361247165615 ) ) ;
#9292=CIRCLE ( 'NONE', #6214, 12.08999999999737440 ) ;
#9295=VECTOR ( 'NONE', #1616, 1000.000000000000000 ) ;
#9296=VECTOR ( 'NONE', #8487, 1000.000000000000000 ) ;
#9306=CARTESIAN_POINT ( 'NONE',  ( -4.072642252455976219, 0.000000000000000000, -12.14623037080101398 ) ) ;
#9307=VERTEX_POINT ( 'NONE', #11526 ) ;
#9310=ORIENTED_EDGE ( 'NONE', *, *, #9812, .T. ) ;
#9313=EDGE_CURVE ( 'NONE', #4866, #10838, #2383, .T. ) ;
#9314=ORIENTED_EDGE ( 'NONE', *, *, #4556, .T. ) ;
#9319=B_SPLINE_CURVE_WITH_KNOTS ( 'NONE', 3,
 ( #1812, #8074, #638, #6009 ),
 .UNSPECIFIED., .F., .F.,
 ( 4, 4 ),
 ( 0.1547128134717859205, 1.000000000000000000 ),
 .UNSPECIFIED. ) ;
#9320=CARTESIAN_POINT ( 'NONE',  ( 8.504652361247167391, 0.000000000000000000, 9.593885948927674434 ) ) ;
#9323=DIRECTION ( 'NONE',  ( -0.000000000000000000, -1.000000000000000000, -0.000000000000000000 ) ) ;
#9324=CARTESIAN_POINT ( 'NONE',  ( 0.000000000000000000, 3.000000000000000000, 0.000000000000000000 ) ) ;
#9325=CARTESIAN_POINT ( 'NONE',  ( -11.52662650599092409, 0.000000000000000000, 3.647599401157420651 ) ) ;
#9343=CARTESIAN_POINT ( 'NONE',  ( -7.065816209474154341, 3.000000000000000000, 10.69794375946289833 ) ) ;
#9345=EDGE_CURVE ( 'NONE', #9927, #10341, #5330, .T. ) ;
#9347=CIRCLE ( 'NONE', #8891, 12.08999999999737263 ) ;
#9349=AXIS2_PLACEMENT_3D ( 'NONE', #10275, #8468, #5102 ) ;
#9350=VERTEX_POINT ( 'NONE', #11393 ) ;
#9354=ORIENTED_EDGE ( 'NONE', *, *, #5934, .F. ) ;
#9367=CARTESIAN_POINT ( 'NONE',  ( -8.922226997226891498, 0.000000000000000000, -8.158551673544284455 ) ) ;
#9369=ORIENTED_EDGE ( 'NONE', *, *, #3703, .T. ) ;
#9372=DIRECTION ( 'NONE',  ( 0.000000000000000000, 0.000000000000000000, -1.000000000000000000 ) ) ;
#9382=CARTESIAN_POINT ( 'NONE',  ( -12.25836857253663759, 0.000000000000000000, -5.784789447945487773 ) ) ;
#9385=ORIENTED_EDGE ( 'NONE', *, *, #6244, .F. ) ;
#9389=ORIENTED_EDGE ( 'NONE', *, *, #8252, .F. ) ;
#9394=CARTESIAN_POINT ( 'NONE',  ( -12.78643498603817896, 3.000000000000000000, 0.7901945867173603144 ) ) ;
#9400=VERTEX_POINT ( 'NONE', #3310 ) ;
#9402=ORIENTED_EDGE ( 'NONE', *, *, #6575, .T. ) ;
#9411=ORIENTED_EDGE ( 'NONE', *, *, #5562, .T. ) ;
#9412=LINE ( 'NONE', #6176, #1587 ) ;
#9413=CYLINDRICAL_SURFACE ( 'NONE', #10626, 14.25000000000000178 ) ;
#9415=CARTESIAN_POINT ( 'NONE',  ( -11.48836750521728867, 0.000000000000000000, -8.430890348300557946 ) ) ;
#9420=LINE ( 'NONE', #887, #7061 ) ;
#9430=B_SPLINE_CURVE_WITH_KNOTS ( 'NONE', 3,
 ( #11506, #12286, #3993, #2003 ),
 .UNSPECIFIED., .F., .F.,
 ( 4, 4 ),
 ( 0.000000000000000000, 0.8452273900860258760 ),
 .UNSPECIFIED. ) ;
#9439=CARTESIAN_POINT ( 'NONE',  ( -8.158551673544545579, 3.000000000000000000, 8.922226997226644585 ) ) ;
#9443=VERTEX_POINT ( 'NONE', #9652 ) ;
#9449=CIRCLE ( 'NONE', #6363, 12.08999999999737085 ) ;
#9450=DIRECTION ( 'NONE',  ( 0.000000000000000000, 0.000000000000000000, 1.000000000000000000 ) ) ;
#9452=EDGE_CURVE ( 'NONE', #10694, #5785, #2211, .T. ) ;
#9454=CARTESIAN_POINT ( 'NONE',  ( -6.506620931068619385, 0.000000000000000000, -10.18979803820057306 ) ) ;
#9455=ORIENTED_EDGE ( 'NONE', *, *, #1183, .T. ) ;
#9457=VERTEX_POINT ( 'NONE', #9787 ) ;
#9461=VERTEX_POINT ( 'NONE', #8744 ) ;
#9467=DIRECTION ( 'NONE',  ( 0.000000000000000000, 0.000000000000000000, -1.000000000000000000 ) ) ;
#9472=CARTESIAN_POINT ( 'NONE',  ( -8.504652361247167391, 3.000000000000000000, -9.593885948927674434 ) ) ;
#9473=VERTEX_POINT ( 'NONE', #9523 ) ;
#9475=LINE ( 'NONE', #9616, #3778 ) ;
#9480=DIRECTION ( 'NONE',  ( 0.000000000000000000, 1.000000000000000000, 0.000000000000000000 ) ) ;
#9484=CARTESIAN_POINT ( 'NONE',  ( -3.647470871583628593, 3.000000000000000000, 11.52666717836884125 ) ) ;
#9485=DIRECTION ( 'NONE',  ( 0.000000000000000000, 0.000000000000000000, 1.000000000000000000 ) ) ;
#9489=ORIENTED_EDGE ( 'NONE', *, *, #8339, .F. ) ;
#9501=CARTESIAN_POINT ( 'NONE',  ( 0.000000000000000000, 3.000000000000000000, 0.000000000000000000 ) ) ;
#9502=DIRECTION ( 'NONE',  ( 0.000000000000000000, 0.000000000000000000, 1.000000000000000000 ) ) ;
#9505=ORIENTED_EDGE ( 'NONE', *, *, #1875, .T. ) ;
#9517=ORIENTED_EDGE ( 'NONE', *, *, #13340, .T. ) ;
#9519=CIRCLE ( 'NONE', #5778, 14.25000000000000178 ) ;
#9522=CIRCLE ( 'NONE', #6872, 14.25000000000000178 ) ;
#9523=CARTESIAN_POINT ( 'NONE',  ( -2.604399508763951321, 0.000000000000000000, 11.80615107470197422 ) ) ;
#9525=CARTESIAN_POINT ( 'NONE',  ( 12.01285915242476499, 3.000000000000000000, -4.000000001073668265 ) ) ;
#9528=FACE_OUTER_BOUND ( 'NONE', #310, .T. ) ;
#9531=CARTESIAN_POINT ( 'NONE',  ( 4.072642252455978884, 0.000000000000000000, 12.14623037080101042 ) ) ;
#9533=ORIENTED_EDGE ( 'NONE', *, *, #8038, .F. ) ;
#9537=CIRCLE ( 'NONE', #6892, 1.499999999686092877 ) ;
#9538=CIRCLE ( 'NONE', #2259, 12.08999999999737440 ) ;
#9548=CARTESIAN_POINT ( 'NONE',  ( 7.712570079660896916, 0.000000000000000000, -11.14709020439929432 ) ) ;
#9549=CARTESIAN_POINT ( 'NONE',  ( 8.914835885878220623, 3.000000000000000000, -11.11702303352196708 ) ) ;
#9550=EDGE_CURVE ( 'NONE', #7235, #10564, #1556, .T. ) ;
#9557=ORIENTED_EDGE ( 'NONE', *, *, #3064, .F. ) ;
#9561=CARTESIAN_POINT ( 'NONE',  ( 2.428572470324196431, 3.000000000000000000, 13.33579367773357127 ) ) ;
#9571=ORIENTED_EDGE ( 'NONE', *, *, #690, .F. ) ;
#9575=CARTESIAN_POINT ( 'NONE',  ( 3.647470871583629926, 3.000000000000000000, -11.52666717836884125 ) ) ;
#9576=DIRECTION ( 'NONE',  ( -0.000000000000000000, -1.000000000000000000, -0.000000000000000000 ) ) ;
#9578=CARTESIAN_POINT ( 'NONE',  ( -4.564691384634503635, 3.000000000000000000, 12.76342233970727769 ) ) ;
#9580=ORIENTED_EDGE ( 'NONE', *, *, #2950, .T. ) ;
#9583=CIRCLE ( 'NONE', #10215, 14.24999999999999822 ) ;
#9584=VERTEX_POINT ( 'NONE', #4694 ) ;
#9603=ORIENTED_EDGE ( 'NONE', *, *, #1455, .T. ) ;
#9605=CARTESIAN_POINT ( 'NONE',  ( 1.557181465540672161, 0.000000000000000000, -14.16466328168010591 ) ) ;
#9609=CARTESIAN_POINT ( 'NONE',  ( 8.504652361247167391, 3.000000000000000000, 9.593885948927674434 ) ) ;
#9610=CARTESIAN_POINT ( 'NONE',  ( 0.000000000000000000, 3.000000000000000000, 0.000000000000000000 ) ) ;
#9615=EDGE_LOOP ( 'NONE', ( #11143, #8855, #2227, #9517 ) ) ;
#9616=CARTESIAN_POINT ( 'NONE',  ( 8.430890348300625448, 3.000000000000000000, 11.48836750521723893 ) ) ;
#9620=CYLINDRICAL_SURFACE ( 'NONE', #5479, 14.25000000000000178 ) ;
#9622=CARTESIAN_POINT ( 'NONE',  ( 5.170206418547656391, 3.000000000000000000, 13.27898586450067064 ) ) ;
#9623=CARTESIAN_POINT ( 'NONE',  ( -8.158551673544545579, 0.000000000000000000, 8.922226997226644585 ) ) ;
#9627=ORIENTED_EDGE ( 'NONE', *, *, #8038, .T. ) ;
#9628=ORIENTED_EDGE ( 'NONE', *, *, #13446, .T. ) ;
#9640=CARTESIAN_POINT ( 'NONE',  ( -3.647470871583628593, 3.000000000000000000, 11.52666717836884125 ) ) ;
#9645=ORIENTED_EDGE ( 'NONE', *, *, #3044, .F. ) ;
#9648=EDGE_LOOP ( 'NONE', ( #11112, #7980, #656, #3688 ) ) ;
#9649=EDGE_CURVE ( 'NONE', #7142, #11145, #9430, .T. ) ;
#9652=CARTESIAN_POINT ( 'NONE',  ( -8.914835885878215294, 0.000000000000000000, 11.11702303352197063 ) ) ;
#9654=CARTESIAN_POINT ( 'NONE',  ( 0.000000000000000000, 3.000000000000000000, 0.000000000000000000 ) ) ;
#9658=DIRECTION ( 'NONE',  ( 1.000000000000000000, 0.000000000000000000, -1.370446048119726253E-16 ) ) ;
#9659=EDGE_LOOP ( 'NONE', ( #1523, #11667, #11698, #4140 ) ) ;
#9660=CARTESIAN_POINT ( 'NONE',  ( 0.000000000000000000, 0.000000000000000000, 0.000000000000000000 ) ) ;
#9664=ORIENTED_EDGE ( 'NONE', *, *, #8769, .T. ) ;
#9667=CARTESIAN_POINT ( 'NONE',  ( -0.7702044561450404059, 0.000000000000000000, 12.79759916868914793 ) ) ;
#9678=ORIENTED_EDGE ( 'NONE', *, *, #6010, .F. ) ;
#9682=CARTESIAN_POINT ( 'NONE',  ( -8.430890348300124515, 3.000000000000000000, 11.48836750521761019 ) ) ;
#9691=ORIENTED_EDGE ( 'NONE', *, *, #788, .T. ) ;
#9692=CIRCLE ( 'NONE', #6619, 12.08999999999737440 ) ;
#9695=CARTESIAN_POINT ( 'NONE',  ( -8.760376775873710997, 3.000000000000000000, 10.34346111134700941 ) ) ;
#9700=AXIS2_PLACEMENT_3D ( 'NONE', #10308, #320, #8560 ) ;
#9704=DIRECTION ( 'NONE',  ( 0.000000000000000000, 0.000000000000000000, -1.000000000000000000 ) ) ;
#9706=FACE_OUTER_BOUND ( 'NONE', #9615, .T. ) ;
#9707=VERTEX_POINT ( 'NONE', #3092 ) ;
#9708=ADVANCED_FACE ( 'NONE', ( #10205 ), #13574, .T. ) ;
#9719=CARTESIAN_POINT ( 'NONE',  ( 2.604399508763947768, 3.000000000000000000, -11.80615107470197778 ) ) ;
#9727=ORIENTED_EDGE ( 'NONE', *, *, #6200, .F. ) ;
#9739=DIRECTION ( 'NONE',  ( -0.000000000000000000, -1.000000000000000000, -0.000000000000000000 ) ) ;
#9741=VECTOR ( 'NONE', #9777, 1000.000000000000000 ) ;
#9758=CARTESIAN_POINT ( 'NONE',  ( 4.577511697546072789, 0.000000000000000000, 12.75843939030335505 ) ) ;
#9759=AXIS2_PLACEMENT_3D ( 'NONE', #13, #12358, #8196 ) ;
#9764=CARTESIAN_POINT ( 'NONE',  ( 31.00000000000000000, 3.000000000000000000, 1.499999998612421725 ) ) ;
#9770=DIRECTION ( 'NONE',  ( -0.000000000000000000, -1.000000000000000000, -0.000000000000000000 ) ) ;
#9777=DIRECTION ( 'NONE',  ( -0.000000000000000000, -1.000000000000000000, -0.000000000000000000 ) ) ;
#9778=EDGE_LOOP ( 'NONE', ( #6008, #5649, #6887, #7891 ) ) ;
#9781=VERTEX_POINT ( 'NONE', #4131 ) ;
#9787=CARTESIAN_POINT ( 'NONE',  ( -3.647470871583628593, 3.000000000000000000, 11.52666717836884125 ) ) ;
#9796=EDGE_LOOP ( 'NONE', ( #11174, #3213, #2644, #2570 ) ) ;
#9800=ORIENTED_EDGE ( 'NONE', *, *, #7671, .T. ) ;
#9801=B_SPLINE_SURFACE_WITH_KNOTS ( 'NONE', 3, 1, ( 
 ( #12298, #13390 ),
 ( #5942, #714 ),
 ( #2840, #9320 ),
 ( #8141, #4913 ) ),
 .UNSPECIFIED., .F., .F., .F.,
 ( 4, 4 ),
 ( 2, 2 ),
 ( 0.000000000000000000, 0.8452273900860258760 ),
 ( 0.000000000000000000, 1.000000000000000000 ),
 .UNSPECIFIED. ) ;
#9805=DIRECTION ( 'NONE',  ( 1.000000000000000000, -0.000000000000000000, -9.145772869372436484E-17 ) ) ;
#9810=DIRECTION ( 'NONE',  ( 0.000000000000000000, 0.000000000000000000, 1.000000000000000000 ) ) ;
#9811=CARTESIAN_POINT ( 'NONE',  ( -2.604399508763951321, 3.000000000000000000, 11.80615107470197422 ) ) ;
#9812=EDGE_CURVE ( 'NONE', #2852, #4189, #9254, .T. ) ;
#9821=CARTESIAN_POINT ( 'NONE',  ( 31.00000000000000000, 0.000000000000000000, -1.073670993220974656E-09 ) ) ;
#9826=EDGE_LOOP ( 'NONE', ( #6902, #2032, #2597, #4665, #3323, #1327, #8044, #7518, #4754, #6362, #9354, #2824, #11156, #1261, #1588, #8538, #1574, #6139, #4614, #324, #1912, #8810, #1663, #2723, #11754, #2926, #8597, #9192, #4361, #13004, #11205, #2996, #4569, #6066, #9126, #2188, #12582, #1557, #5873, #5872, #12558, #8725, #4759, #4223, #3300, #13373, #4346, #12894, #6241, #11089, #4578, #5629, #2166, #3421, #2539, #4483, #1745, #9533, #8550, #4478, #6717, #7447, #7385, #9489, #10871, #1775, #12505, #12579, #7566, #10967, #2238, #5760, #12340, #10689, #3920, #6703, #849, #8153, #7619, #9571, #8170, #6825, #13569, #5577, #831, #9678, #6564, #11977, #4802, #6034, #3459 ) ) ;
#9828=CARTESIAN_POINT ( 'NONE',  ( -8.158551673544545579, 3.000000000000000000, 8.922226997226644585 ) ) ;
#9831=LINE ( 'NONE', #2469, #11650 ) ;
#9834=CARTESIAN_POINT ( 'NONE',  ( -8.922226997226788470, 0.000000000000000000, -8.158551673544387484 ) ) ;
#9835=CARTESIAN_POINT ( 'NONE',  ( 0.000000000000000000, 3.000000000000000000, 0.000000000000000000 ) ) ;
#9836=CARTESIAN_POINT ( 'NONE',  ( 8.482622935103764306, 0.000000000000000000, -9.600126836553261711 ) ) ;
#9838=VERTEX_POINT ( 'NONE', #6583 ) ;
#9839=CYLINDRICAL_SURFACE ( 'NONE', #12620, 14.25000000000000000 ) ;
#9840=VERTEX_POINT ( 'NONE', #9952 ) ;
#9841=ORIENTED_EDGE ( 'NONE', *, *, #5889, .T. ) ;
#9845=EDGE_LOOP ( 'NONE', ( #8721, #1944, #10981, #2966 ) ) ;
#9852=CYLINDRICAL_SURFACE ( 'NONE', #1997, 1.499999999686092877 ) ;
#9853=CARTESIAN_POINT ( 'NONE',  ( 2.161962830978694683, 0.000000000000000000, -14.08504230442587790 ) ) ;
#9858=DIRECTION ( 'NONE',  ( 0.000000000000000000, 1.000000000000000000, 0.000000000000000000 ) ) ;
#9859=ORIENTED_EDGE ( 'NONE', *, *, #6920, .T. ) ;
#9863=CARTESIAN_POINT ( 'NONE',  ( 12.90250726680438476, 3.000000000000000000, 4.728042766759046778 ) ) ;
#9866=ADVANCED_FACE ( 'NONE', ( #10861 ), #8728, .F. ) ;
#9868=CARTESIAN_POINT ( 'NONE',  ( 10.69794375946289655, 3.000000000000000000, 7.065816209474157006 ) ) ;
#9869=DIRECTION ( 'NONE',  ( 0.000000000000000000, 0.000000000000000000, 1.000000000000000000 ) ) ;
#9871=B_SPLINE_CURVE_WITH_KNOTS ( 'NONE', 3,
 ( #1976, #1013, #9343, #1073 ),
 .UNSPECIFIED., .F., .F.,
 ( 4, 4 ),
 ( 0.000000000000000000, 0.8452273900860258760 ),
 .UNSPECIFIED. ) ;
#9872=CARTESIAN_POINT ( 'NONE',  ( -12.79759916868914615, 0.000000000000000000, -0.7702044561450367421 ) ) ;
#9874=VERTEX_POINT ( 'NONE', #6332 ) ;
#9886=DIRECTION ( 'NONE',  ( 0.000000000000000000, 0.000000000000000000, 1.000000000000000000 ) ) ;
#9890=ADVANCED_FACE ( 'NONE', ( #331 ), #7684, .T. ) ;
#9891=VERTEX_POINT ( 'NONE', #5547 ) ;
#9897=DIRECTION ( 'NONE',  ( 0.000000000000000000, 1.000000000000000000, 0.000000000000000000 ) ) ;
#9902=CIRCLE ( 'NONE', #3305, 14.25000000000000178 ) ;
#9903=DIRECTION ( 'NONE',  ( 0.000000000000000000, 0.000000000000000000, -1.000000000000000000 ) ) ;
#9905=DIRECTION ( 'NONE',  ( -0.000000000000000000, -1.000000000000000000, -0.000000000000000000 ) ) ;
#9912=CIRCLE ( 'NONE', #12790, 14.25000000000000178 ) ;
#9913=ORIENTED_EDGE ( 'NONE', *, *, #5607, .F. ) ;
#9914=CIRCLE ( 'NONE', #5523, 14.25000000000000000 ) ;
#9918=CARTESIAN_POINT ( 'NONE',  ( 0.000000000000000000, 0.000000000000000000, 0.000000000000000000 ) ) ;
#9920=CARTESIAN_POINT ( 'NONE',  ( -0.7901945867173586491, 3.000000000000000000, -12.78643498603818074 ) ) ;
#9923=CARTESIAN_POINT ( 'NONE',  ( 5.170206418547656391, 3.000000000000000000, 13.27898586450067064 ) ) ;
#9927=VERTEX_POINT ( 'NONE', #1704 ) ;
#9931=CARTESIAN_POINT ( 'NONE',  ( -13.33579367773357482, 3.000000000000000000, 2.428572470324200427 ) ) ;
#9937=CARTESIAN_POINT ( 'NONE',  ( -12.07793442604884682, 0.000000000000000000, 0.5400000000005513723 ) ) ;
#9939=CARTESIAN_POINT ( 'NONE',  ( -5.170206418547658167, 3.000000000000000000, -13.27898586450066887 ) ) ;
#9943=ORIENTED_EDGE ( 'NONE', *, *, #3970, .T. ) ;
#9947=B_SPLINE_SURFACE_WITH_KNOTS ( 'NONE', 3, 1, ( 
 ( #7805, #5734 ),
 ( #9931, #509 ),
 ( #1955, #796 ),
 ( #6145, #9243 ) ),
 .UNSPECIFIED., .F., .F., .F.,
 ( 4, 4 ),
 ( 2, 2 ),
 ( 0.000000000000000000, 0.8452273900860258760 ),
 ( 0.000000000000000000, 1.000000000000000000 ),
 .UNSPECIFIED. ) ;
#9949=CARTESIAN_POINT ( 'NONE',  ( 5.797378255456016483, 3.000000000000000000, 12.25282671965375592 ) ) ;
#9952=CARTESIAN_POINT ( 'NONE',  ( 11.11702303352194043, 3.000000000000000000, -8.914835885878249044 ) ) ;
#9953=AXIS2_PLACEMENT_3D ( 'NONE', #12102, #2653, #4858 ) ;
#9958=CARTESIAN_POINT ( 'NONE',  ( 12.89546620003432764, 3.000000000000000000, -4.733530556166651415 ) ) ;
#9960=DIRECTION ( 'NONE',  ( 0.000000000000000000, 1.000000000000000000, 0.000000000000000000 ) ) ;
#9963=VERTEX_POINT ( 'NONE', #12390 ) ;
#9964=VERTEX_POINT ( 'NONE', #10161 ) ;
#9967=AXIS2_PLACEMENT_3D ( 'NONE', #8015, #12235, #2782 ) ;
#9968=CIRCLE ( 'NONE', #3155, 14.25000000000000000 ) ;
#9977=DIRECTION ( 'NONE',  ( -0.000000000000000000, -1.000000000000000000, -0.000000000000000000 ) ) ;
#9983=EDGE_LOOP ( 'NONE', ( #9841, #10214, #2256, #6532 ) ) ;
#9989=CARTESIAN_POINT ( 'NONE',  ( -13.27898586450070084, 0.000000000000000000, -5.170206418547588001 ) ) ;
#9994=CARTESIAN_POINT ( 'NONE',  ( -10.72979803820123479, 0.000000000000000000, -5.571313494980285164 ) ) ;
#9996=ORIENTED_EDGE ( 'NONE', *, *, #364, .T. ) ;
#9998=CARTESIAN_POINT ( 'NONE',  ( 4.072642252455978884, 3.000000000000000000, 12.14623037080101042 ) ) ;
#10007=AXIS2_PLACEMENT_3D ( 'NONE', #6754, #3381, #5712 ) ;
#10008=AXIS2_PLACEMENT_3D ( 'NONE', #7579, #2271, #9704 ) ;
#10012=FACE_OUTER_BOUND ( 'NONE', #7121, .T. ) ;
#10013=CARTESIAN_POINT ( 'NONE',  ( 8.430890348300625448, 3.000000000000000000, 11.48836750521723893 ) ) ;
#10016=CARTESIAN_POINT ( 'NONE',  ( 11.13895890373327724, 3.000000000000000000, -7.723663868796764476 ) ) ;
#10019=VERTEX_POINT ( 'NONE', #6932 ) ;
#10021=EDGE_CURVE ( 'NONE', #9046, #2645, #7334, .T. ) ;
#10022=VERTEX_POINT ( 'NONE', #6856 ) ;
#10023=B_SPLINE_CURVE_WITH_KNOTS ( 'NONE', 3,
 ( #370, #302, #12766, #4561 ),
 .UNSPECIFIED., .F., .F.,
 ( 4, 4 ),
 ( 0.000000000000000000, 0.8452273900860258760 ),
 .UNSPECIFIED. ) ;
#10027=EDGE_LOOP ( 'NONE', ( #8106, #2466, #1848, #13202 ) ) ;
#10028=EDGE_CURVE ( 'NONE', #2208, #10549, #4794, .T. ) ;
#10032=DIRECTION ( 'NONE',  ( 0.000000000000000000, 1.000000000000000000, 0.000000000000000000 ) ) ;
#10050=VERTEX_POINT ( 'NONE', #5266 ) ;
#10051=DIRECTION ( 'NONE',  ( 0.000000000000000000, 0.000000000000000000, -1.000000000000000000 ) ) ;
#10053=B_SPLINE_SURFACE_WITH_KNOTS ( 'NONE', 3, 1, ( 
 ( #5698, #10560 ),
 ( #11600, #2155 ),
 ( #10634, #3384 ),
 ( #6351, #7597 ) ),
 .UNSPECIFIED., .F., .F., .F.,
 ( 4, 4 ),
 ( 2, 2 ),
 ( 0.1547128134717859205, 1.000000000000000000 ),
 ( 0.000000000000000000, 1.000000000000000000 ),
 .UNSPECIFIED. ) ;
#10054=ORIENTED_EDGE ( 'NONE', *, *, #6502, .T. ) ;
#10055=CARTESIAN_POINT ( 'NONE',  ( 7.065816209474156118, 0.000000000000000000, -10.69794375946289833 ) ) ;
#10059=CARTESIAN_POINT ( 'NONE',  ( -10.18987059060247624, 0.000000000000000000, -6.506507307819711095 ) ) ;
#10072=CARTESIAN_POINT ( 'NONE',  ( -10.18979803820068675, 0.000000000000000000, 6.506620931068438196 ) ) ;
#10074=ORIENTED_EDGE ( 'NONE', *, *, #7324, .T. ) ;
#10078=CARTESIAN_POINT ( 'NONE',  ( -12.25282671965375236, 3.000000000000000000, 5.797378255456025364 ) ) ;
#10082=LINE ( 'NONE', #3608, #13226 ) ;
#10085=ORIENTED_EDGE ( 'NONE', *, *, #5916, .F. ) ;
#10087=VERTEX_POINT ( 'NONE', #8232 ) ;
#10093=DIRECTION ( 'NONE',  ( 0.000000000000000000, 0.000000000000000000, 1.000000000000000000 ) ) ;
#10094=CYLINDRICAL_SURFACE ( 'NONE', #7147, 12.08999999999737618 ) ;
#10096=EDGE_CURVE ( 'NONE', #3304, #10338, #10410, .T. ) ;
#10103=CARTESIAN_POINT ( 'NONE',  ( 13.04554897075799502, 0.000000000000000000, 5.733772933379473358 ) ) ;
#10111=ORIENTED_EDGE ( 'NONE', *, *, #5610, .F. ) ;
#10112=FACE_OUTER_BOUND ( 'NONE', #1500, .T. ) ;
#10120=CARTESIAN_POINT ( 'NONE',  ( -6.506507307819711095, 3.000000000000000000, 10.18987059060247624 ) ) ;
#10126=AXIS2_PLACEMENT_3D ( 'NONE', #9324, #3878, #1055 ) ;
#10130=CARTESIAN_POINT ( 'NONE',  ( 2.428572470324196431, 3.000000000000000000, 13.33579367773357127 ) ) ;
#10132=ORIENTED_EDGE ( 'NONE', *, *, #4323, .T. ) ;
#10135=ORIENTED_EDGE ( 'NONE', *, *, #151, .T. ) ;
#10138=B_SPLINE_SURFACE_WITH_KNOTS ( 'NONE', 3, 1, ( 
 ( #659, #6719 ),
 ( #11962, #2791 ),
 ( #7001, #11197 ),
 ( #2522, #10922 ) ),
 .UNSPECIFIED., .F., .F., .F.,
 ( 4, 4 ),
 ( 2, 2 ),
 ( 0.1547128134717859205, 1.000000000000000000 ),
 ( 0.000000000000000000, 1.000000000000000000 ),
 .UNSPECIFIED. ) ;
#10140=ORIENTED_EDGE ( 'NONE', *, *, #364, .F. ) ;
#10145=CARTESIAN_POINT ( 'NONE',  ( 11.48836750521724070, 3.000000000000000000, -8.430890348300621895 ) ) ;
#10161=CARTESIAN_POINT ( 'NONE',  ( -11.48836750521723893, 0.000000000000000000, 8.430890348300625448 ) ) ;
#10166=VECTOR ( 'NONE', #9739, 1000.000000000000000 ) ;
#10167=CARTESIAN_POINT ( 'NONE',  ( -14.16466328168010769, 3.000000000000000000, -1.557181465540670384 ) ) ;
#10168=CARTESIAN_POINT ( 'NONE',  ( -0.5398653231797316820, 3.000000000000000000, 12.07794044664754018 ) ) ;
#10170=ORIENTED_EDGE ( 'NONE', *, *, #5493, .T. ) ;
#10173=ORIENTED_EDGE ( 'NONE', *, *, #1148, .T. ) ;
#10178=DIRECTION ( 'NONE',  ( 0.000000000000000000, 0.000000000000000000, 1.000000000000000000 ) ) ;
#10181=CARTESIAN_POINT ( 'NONE',  ( -11.80615107470197778, 3.000000000000000000, -2.604399508763947768 ) ) ;
#10182=LINE ( 'NONE', #11363, #6384 ) ;
#10186=ORIENTED_EDGE ( 'NONE', *, *, #6999, .F. ) ;
#10197=EDGE_CURVE ( 'NONE', #9838, #9046, #4164, .T. ) ;
#10205=FACE_OUTER_BOUND ( 'NONE', #2036, .T. ) ;
#10208=LINE ( 'NONE', #7921, #2503 ) ;
#10211=DIRECTION ( 'NONE',  ( 0.000000000000000000, 0.000000000000000000, 1.000000000000000000 ) ) ;
#10214=ORIENTED_EDGE ( 'NONE', *, *, #1270, .F. ) ;
#10215=AXIS2_PLACEMENT_3D ( 'NONE', #8236, #13413, #10375 ) ;
#10218=FACE_OUTER_BOUND ( 'NONE', #8289, .T. ) ;
#10220=ADVANCED_FACE ( 'NONE', ( #2040 ), #939, .T. ) ;
#10221=DIRECTION ( 'NONE',  ( -0.000000000000000000, -1.000000000000000000, -0.000000000000000000 ) ) ;
#10222=CARTESIAN_POINT ( 'NONE',  ( 11.13895890373327724, 3.000000000000000000, -7.723663868796764476 ) ) ;
#10224=CARTESIAN_POINT ( 'NONE',  ( 0.000000000000000000, 0.000000000000000000, 0.000000000000000000 ) ) ;
#10228=CIRCLE ( 'NONE', #1861, 14.25000000000000355 ) ;
#10233=DIRECTION ( 'NONE',  ( -0.000000000000000000, -1.000000000000000000, -0.000000000000000000 ) ) ;
#10234=ORIENTED_EDGE ( 'NONE', *, *, #6115, .T. ) ;
#10235=ORIENTED_EDGE ( 'NONE', *, *, #10488, .T. ) ;
#10237=AXIS2_PLACEMENT_3D ( 'NONE', #11603, #5391, #9658 ) ;
#10238=EDGE_CURVE ( 'NONE', #5441, #9874, #7410, .T. ) ;
#10244=DIRECTION ( 'NONE',  ( 0.000000000000000000, 1.000000000000000000, 0.000000000000000000 ) ) ;
#10246=MECHANICAL_DESIGN_GEOMETRIC_PRESENTATION_REPRESENTATION('',(#8259),#4523);
#10256=FACE_OUTER_BOUND ( 'NONE', #6810, .T. ) ;
#10259=FACE_OUTER_BOUND ( 'NONE', #12751, .T. ) ;
#10268=ORIENTED_EDGE ( 'NONE', *, *, #5555, .F. ) ;
#10273=CYLINDRICAL_SURFACE ( 'NONE', #13293, 14.25000000000000178 ) ;
#10275=CARTESIAN_POINT ( 'NONE',  ( 0.000000000000000000, 3.000000000000000000, 0.000000000000000000 ) ) ;
#10279=ORIENTED_EDGE ( 'NONE', *, *, #10901, .T. ) ;
#10286=CARTESIAN_POINT ( 'NONE',  ( 10.67828022838850366, 3.000000000000000000, -7.077546079049271022 ) ) ;
#10288=DIRECTION ( 'NONE',  ( 0.000000000000000000, 0.000000000000000000, 1.000000000000000000 ) ) ;
#10289=B_SPLINE_CURVE_WITH_KNOTS ( 'NONE', 3,
 ( #1017, #3136, #817, #7349 ),
 .UNSPECIFIED., .F., .F.,
 ( 4, 4 ),
 ( 0.000000000000000000, 0.8452273900860258760 ),
 .UNSPECIFIED. ) ;
#10295=FACE_OUTER_BOUND ( 'NONE', #3061, .T. ) ;
#10297=ORIENTED_EDGE ( 'NONE', *, *, #10096, .F. ) ;
#10299=ORIENTED_EDGE ( 'NONE', *, *, #7201, .T. ) ;
#10307=CARTESIAN_POINT ( 'NONE',  ( 0.000000000000000000, 3.000000000000000000, 0.000000000000000000 ) ) ;
#10308=CARTESIAN_POINT ( 'NONE',  ( 0.000000000000000000, 3.000000000000000000, 0.000000000000000000 ) ) ;
#10311=CARTESIAN_POINT ( 'NONE',  ( -1.105736515254454044, 3.000000000000000000, 13.50994833511691340 ) ) ;
#10318=CARTESIAN_POINT ( 'NONE',  ( 0.000000000000000000, 3.000000000000000000, 0.000000000000000000 ) ) ;
#10321=ADVANCED_FACE ( 'NONE', ( #4574 ), #8835, .F. ) ;
#10338=VERTEX_POINT ( 'NONE', #11122 ) ;
#10339=DIRECTION ( 'NONE',  ( 0.000000000000000000, 1.000000000000000000, 0.000000000000000000 ) ) ;
#10341=VERTEX_POINT ( 'NONE', #13181 ) ;
#10348=DIRECTION ( 'NONE',  ( 0.000000000000000000, 1.000000000000000000, 0.000000000000000000 ) ) ;
#10349=CARTESIAN_POINT ( 'NONE',  ( 0.000000000000000000, 0.000000000000000000, 0.000000000000000000 ) ) ;
#10351=CARTESIAN_POINT ( 'NONE',  ( -5.733772933379472470, 3.000000000000000000, 13.04554897075799502 ) ) ;
#10353=DIRECTION ( 'NONE',  ( 0.000000000000000000, 0.000000000000000000, 1.000000000000000000 ) ) ;
#10354=DIRECTION ( 'NONE',  ( 0.000000000000000000, 1.000000000000000000, 0.000000000000000000 ) ) ;
#10356=CARTESIAN_POINT ( 'NONE',  ( -2.161962830978783057, 0.000000000000000000, -14.08504230442586369 ) ) ;
#10359=AXIS2_PLACEMENT_3D ( 'NONE', #9821, #4451, #6585 ) ;
#10361=VERTEX_POINT ( 'NONE', #10013 ) ;
#10375=DIRECTION ( 'NONE',  ( 0.000000000000000000, 0.000000000000000000, 1.000000000000000000 ) ) ;
#10378=VECTOR ( 'NONE', #4073, 1000.000000000000000 ) ;
#10387=AXIS2_PLACEMENT_3D ( 'NONE', #11154, #11993, #555 ) ;
#10388=CARTESIAN_POINT ( 'NONE',  ( -6.506620931068619385, 3.000000000000000000, -10.18979803820057306 ) ) ;
#10393=CARTESIAN_POINT ( 'NONE',  ( 2.604399508763944660, 0.000000000000000000, -11.80615107470197600 ) ) ;
#10396=EDGE_LOOP ( 'NONE', ( #8927, #129, #807, #2160 ) ) ;
#10402=EDGE_CURVE ( 'NONE', #10019, #3932, #751, .T. ) ;
#10403=DIRECTION ( 'NONE',  ( 0.000000000000000000, 0.000000000000000000, -1.000000000000000000 ) ) ;
#10406=CARTESIAN_POINT ( 'NONE',  ( 0.000000000000000000, 3.000000000000000000, 0.000000000000000000 ) ) ;
#10410=CIRCLE ( 'NONE', #4462, 14.25000000000000178 ) ;
#10416=ORIENTED_EDGE ( 'NONE', *, *, #5562, .F. ) ;
#10426=CARTESIAN_POINT ( 'NONE',  ( 8.922226997226882617, 0.000000000000000000, 8.158551673544282679 ) ) ;
#10430=CYLINDRICAL_SURFACE ( 'NONE', #12799, 14.25000000000000000 ) ;
#10433=DIRECTION ( 'NONE',  ( -0.000000000000000000, -1.000000000000000000, -0.000000000000000000 ) ) ;
#10434=CIRCLE ( 'NONE', #4487, 1.500000000000000222 ) ;
#10436=ORIENTED_EDGE ( 'NONE', *, *, #4706, .T. ) ;
#10439=VERTEX_POINT ( 'NONE', #5737 ) ;
#10443=VECTOR ( 'NONE', #5420, 1000.000000000000000 ) ;
#10452=ORIENTED_EDGE ( 'NONE', *, *, #5148, .F. ) ;
#10460=CARTESIAN_POINT ( 'NONE',  ( -5.170206418547658167, 3.000000000000000000, -13.27898586450066887 ) ) ;
#10466=DIRECTION ( 'NONE',  ( 0.000000000000000000, 0.000000000000000000, 1.000000000000000000 ) ) ;
#10468=CARTESIAN_POINT ( 'NONE',  ( 13.04554897075799502, 3.000000000000000000, 5.733772933379473358 ) ) ;
#10469=EDGE_CURVE ( 'NONE', #4442, #3224, #11076, .T. ) ;
#10470=ORIENTED_EDGE ( 'NONE', *, *, #10486, .T. ) ;
#10481=DIRECTION ( 'NONE',  ( -0.000000000000000000, -1.000000000000000000, -0.000000000000000000 ) ) ;
#10486=EDGE_CURVE ( 'NONE', #11304, #5111, #8905, .T. ) ;
#10487=ORIENTED_EDGE ( 'NONE', *, *, #11889, .T. ) ;
#10488=EDGE_CURVE ( 'NONE', #5675, #3853, #9537, .T. ) ;
#10491=ORIENTED_EDGE ( 'NONE', *, *, #13345, .F. ) ;
#10493=DIRECTION ( 'NONE',  ( 0.000000000000000000, 0.000000000000000000, 1.000000000000000000 ) ) ;
#10495=CARTESIAN_POINT ( 'NONE',  ( 0.000000000000000000, 3.000000000000000000, 0.000000000000000000 ) ) ;
#10497=CARTESIAN_POINT ( 'NONE',  ( -12.07793442604884682, 3.000000000000000000, 0.5400000000005513723 ) ) ;
#10511=CARTESIAN_POINT ( 'NONE',  ( 0.000000000000000000, 3.000000000000000000, 0.000000000000000000 ) ) ;
#10517=VERTEX_POINT ( 'NONE', #9325 ) ;
#10520=FACE_OUTER_BOUND ( 'NONE', #4772, .T. ) ;
#10526=EDGE_CURVE ( 'NONE', #6360, #12046, #7397, .T. ) ;
#10529=CARTESIAN_POINT ( 'NONE',  ( 13.04554897075799502, 3.000000000000000000, 5.733772933379473358 ) ) ;
#10533=ORIENTED_EDGE ( 'NONE', *, *, #113, .T. ) ;
#10534=CYLINDRICAL_SURFACE ( 'NONE', #13040, 12.08999999999737440 ) ;
#10536=DIRECTION ( 'NONE',  ( 0.000000000000000000, 1.000000000000000000, 0.000000000000000000 ) ) ;
#10545=CARTESIAN_POINT ( 'NONE',  ( 11.48836750521724070, 0.000000000000000000, -8.430890348300621895 ) ) ;
#10549=VERTEX_POINT ( 'NONE', #12638 ) ;
#10550=EDGE_CURVE ( 'NONE', #4058, #1501, #2716, .T. ) ;
#10553=ORIENTED_EDGE ( 'NONE', *, *, #3633, .T. ) ;
#10560=CARTESIAN_POINT ( 'NONE',  ( -2.604399508763953985, 0.000000000000000000, 11.80615107470197778 ) ) ;
#10563=CARTESIAN_POINT ( 'NONE',  ( 31.00000000000000000, 3.000000000000000000, 1.499999998612421725 ) ) ;
#10564=VERTEX_POINT ( 'NONE', #12512 ) ;
#10566=ORIENTED_EDGE ( 'NONE', *, *, #10028, .F. ) ;
#10582=CARTESIAN_POINT ( 'NONE',  ( -5.170206418547586225, 3.000000000000000000, 13.27898586450069907 ) ) ;
#10586=VECTOR ( 'NONE', #13022, 1000.000000000000000 ) ;
#10587=VECTOR ( 'NONE', #13131, 1000.000000000000000 ) ;
#10588=ORIENTED_EDGE ( 'NONE', *, *, #2874, .T. ) ;
#10592=DIRECTION ( 'NONE',  ( -0.000000000000000000, -1.000000000000000000, -0.000000000000000000 ) ) ;
#10594=DIRECTION ( 'NONE',  ( 0.000000000000000000, 1.000000000000000000, 0.000000000000000000 ) ) ;
#10597=EDGE_LOOP ( 'NONE', ( #9627, #11226, #466, #5973 ) ) ;
#10610=CARTESIAN_POINT ( 'NONE',  ( 0.000000000000000000, 0.000000000000000000, 0.000000000000000000 ) ) ;
#10612=CARTESIAN_POINT ( 'NONE',  ( 2.604531154829233586, 0.000000000000000000, 11.80612203322752585 ) ) ;
#10614=ORIENTED_EDGE ( 'NONE', *, *, #6136, .F. ) ;
#10616=CARTESIAN_POINT ( 'NONE',  ( -12.79759916868914615, 3.000000000000000000, -0.7702044561450367421 ) ) ;
#10617=ORIENTED_EDGE ( 'NONE', *, *, #5906, .F. ) ;
#10619=AXIS2_PLACEMENT_3D ( 'NONE', #3392, #1262, #5454 ) ;
#10626=AXIS2_PLACEMENT_3D ( 'NONE', #6177, #13556, #2116 ) ;
#10634=CARTESIAN_POINT ( 'NONE',  ( -2.414978278956346092, 3.000000000000000000, 13.33788847341978467 ) ) ;
#10636=CARTESIAN_POINT ( 'NONE',  ( 10.34346111134700585, 3.000000000000000000, 8.760376775873716326 ) ) ;
#10644=ADVANCED_FACE ( 'NONE', ( #3313 ), #6762, .F. ) ;
#10646=ORIENTED_EDGE ( 'NONE', *, *, #10028, .T. ) ;
#10654=CARTESIAN_POINT ( 'NONE',  ( 6.506620931068707314, 0.000000000000000000, 10.18979803820051622 ) ) ;
#10657=ORIENTED_EDGE ( 'NONE', *, *, #4160, .T. ) ;
#10658=EDGE_CURVE ( 'NONE', #1111, #13326, #2291, .T. ) ;
#10659=CARTESIAN_POINT ( 'NONE',  ( 11.11702303352196708, 3.000000000000000000, 8.914835885878218846 ) ) ;
#10667=CARTESIAN_POINT ( 'NONE',  ( -0.5400000000007666445, 3.000000000000000000, -12.07793442604883793 ) ) ;
#10680=SURFACE_SIDE_STYLE ('',( #6471 ) ) ;
#10682=DIRECTION ( 'NONE',  ( 0.000000000000000000, 1.000000000000000000, 0.000000000000000000 ) ) ;
#10687=ORIENTED_EDGE ( 'NONE', *, *, #5610, .T. ) ;
#10688=EDGE_LOOP ( 'NONE', ( #10951, #7664, #2806, #12827 ) ) ;
#10689=ORIENTED_EDGE ( 'NONE', *, *, #8101, .F. ) ;
#10692=ORIENTED_EDGE ( 'NONE', *, *, #5747, .T. ) ;
#10694=VERTEX_POINT ( 'NONE', #13591 ) ;
#10698=CARTESIAN_POINT ( 'NONE',  ( 10.72979803820131472, 3.000000000000000000, 5.571313494980131509 ) ) ;
#10702=CARTESIAN_POINT ( 'NONE',  ( 0.000000000000000000, 3.000000000000000000, 0.000000000000000000 ) ) ;
#10716=DIRECTION ( 'NONE',  ( 0.000000000000000000, 0.000000000000000000, 1.000000000000000000 ) ) ;
#10718=EDGE_CURVE ( 'NONE', #12859, #1247, #12905, .T. ) ;
#10719=EDGE_LOOP ( 'NONE', ( #8615, #7083, #7102, #9081 ) ) ;
#10722=B_SPLINE_SURFACE_WITH_KNOTS ( 'NONE', 3, 1, ( 
 ( #2620, #4827 ),
 ( #5867, #6822 ),
 ( #7853, #11238 ),
 ( #3864, #1807 ) ),
 .UNSPECIFIED., .F., .F., .F.,
 ( 4, 4 ),
 ( 2, 2 ),
 ( 0.1547128134717859205, 1.000000000000000000 ),
 ( 0.000000000000000000, 1.000000000000000000 ),
 .UNSPECIFIED. ) ;
#10723=ORIENTED_EDGE ( 'NONE', *, *, #6420, .T. ) ;
#10727=LINE ( 'NONE', #7424, #7493 ) ;
#10728=DIRECTION ( 'NONE',  ( 0.000000000000000000, 0.000000000000000000, 1.000000000000000000 ) ) ;
#10736=CARTESIAN_POINT ( 'NONE',  ( -8.922136023539609440, 0.000000000000000000, 8.158651161643900807 ) ) ;
#10737=ORIENTED_EDGE ( 'NONE', *, *, #12101, .T. ) ;
#10742=DIRECTION ( 'NONE',  ( 0.000000000000000000, 1.000000000000000000, 0.000000000000000000 ) ) ;
#10747=LINE ( 'NONE', #159, #9741 ) ;
#10752=CARTESIAN_POINT ( 'NONE',  ( -5.170206418547117266, 0.000000000000000000, 13.27898586450088203 ) ) ;
#10755=DIRECTION ( 'NONE',  ( -0.000000000000000000, -1.000000000000000000, -0.000000000000000000 ) ) ;
#10757=CARTESIAN_POINT ( 'NONE',  ( 12.01285915242476499, 3.000000000000000000, -4.000000001073668265 ) ) ;
#10760=DIRECTION ( 'NONE',  ( -0.000000000000000000, -1.000000000000000000, -0.000000000000000000 ) ) ;
#10764=ORIENTED_EDGE ( 'NONE', *, *, #6899, .T. ) ;
#10766=CIRCLE ( 'NONE', #7039, 14.25000000000000000 ) ;
#10767=ADVANCED_FACE ( 'NONE', ( #5929 ), #10722, .F. ) ;
#10774=FACE_OUTER_BOUND ( 'NONE', #10597, .T. ) ;
#10775=CIRCLE ( 'NONE', #12137, 14.25000000000000000 ) ;
#10778=CARTESIAN_POINT ( 'NONE',  ( 9.600126836553261711, 3.000000000000000000, 8.482622935103766082 ) ) ;
#10779=EDGE_CURVE ( 'NONE', #9927, #3195, #10208, .T. ) ;
#10780=VERTEX_POINT ( 'NONE', #13236 ) ;
#10784=CARTESIAN_POINT ( 'NONE',  ( 0.000000000000000000, 3.000000000000000000, 0.000000000000000000 ) ) ;
#10789=CARTESIAN_POINT ( 'NONE',  ( -5.797378255456022700, 3.000000000000000000, -12.25282671965375592 ) ) ;
#10791=ORIENTED_EDGE ( 'NONE', *, *, #508, .T. ) ;
#10793=VERTEX_POINT ( 'NONE', #11026 ) ;
#10799=EDGE_LOOP ( 'NONE', ( #13038, #12892, #12839, #5304 ) ) ;
#10804=CARTESIAN_POINT ( 'NONE',  ( -10.72979803820123479, 3.000000000000000000, -5.571313494980285164 ) ) ;
#10806=CYLINDRICAL_SURFACE ( 'NONE', #5834, 14.25000000000000000 ) ;
#10807=ORIENTED_EDGE ( 'NONE', *, *, #2194, .T. ) ;
#10812=VERTEX_POINT ( 'NONE', #7997 ) ;
#10821=EDGE_CURVE ( 'NONE', #9964, #8384, #3163, .T. ) ;
#10829=CARTESIAN_POINT ( 'NONE',  ( 8.922226997226882617, 3.000000000000000000, 8.158551673544282679 ) ) ;
#10837=AXIS2_PLACEMENT_3D ( 'NONE', #2762, #775, #10403 ) ;
#10838=VERTEX_POINT ( 'NONE', #13168 ) ;
#10849=FACE_OUTER_BOUND ( 'NONE', #9659, .T. ) ;
#10851=ORIENTED_EDGE ( 'NONE', *, *, #12173, .F. ) ;
#10860=AXIS2_PLACEMENT_3D ( 'NONE', #1920, #7154, #11414 ) ;
#10861=FACE_OUTER_BOUND ( 'NONE', #1760, .T. ) ;
#10863=DIRECTION ( 'NONE',  ( -0.000000000000000000, -1.000000000000000000, -0.000000000000000000 ) ) ;
#10865=EDGE_CURVE ( 'NONE', #8366, #1810, #6463, .T. ) ;
#10867=ADVANCED_FACE ( 'NONE', ( #5234 ), #2973, .T. ) ;
#10871=ORIENTED_EDGE ( 'NONE', *, *, #6899, .F. ) ;
#10880=CARTESIAN_POINT ( 'NONE',  ( -10.34346111134701118, 0.000000000000000000, -8.760376775873707444 ) ) ;
#10884=CARTESIAN_POINT ( 'NONE',  ( 8.158551673544288008, 3.000000000000000000, -8.922226997226886169 ) ) ;
#10887=ORIENTED_EDGE ( 'NONE', *, *, #6101, .F. ) ;
#10901=EDGE_CURVE ( 'NONE', #4277, #9276, #13379, .T. ) ;
#10904=CARTESIAN_POINT ( 'NONE',  ( -12.75843939030334795, 0.000000000000000000, 4.577511697546079006 ) ) ;
#10909=DIRECTION ( 'NONE',  ( -0.000000000000000000, -1.000000000000000000, -0.000000000000000000 ) ) ;
#10910=CARTESIAN_POINT ( 'NONE',  ( 5.571433138827823761, 0.000000000000000000, 10.72973591378220704 ) ) ;
#10911=DIRECTION ( 'NONE',  ( -0.000000000000000000, -1.000000000000000000, -0.000000000000000000 ) ) ;
#10914=CARTESIAN_POINT ( 'NONE',  ( 0.000000000000000000, 0.000000000000000000, 0.000000000000000000 ) ) ;
#10919=B_SPLINE_CURVE_WITH_KNOTS ( 'NONE', 3,
 ( #4908, #6980, #12225, #11323 ),
 .UNSPECIFIED., .F., .F.,
 ( 4, 4 ),
 ( 0.000000000000000000, 0.8452273900860258760 ),
 .UNSPECIFIED. ) ;
#10922=CARTESIAN_POINT ( 'NONE',  ( -8.914835885878215294, 0.000000000000000000, 11.11702303352197063 ) ) ;
#10925=CARTESIAN_POINT ( 'NONE',  ( -9.600126836553261711, 3.000000000000000000, -8.482622935103767858 ) ) ;
#10928=CARTESIAN_POINT ( 'NONE',  ( 12.89546620003432764, 0.000000000000000000, -4.733530556166651415 ) ) ;
#10933=ORIENTED_EDGE ( 'NONE', *, *, #8252, .T. ) ;
#10937=EDGE_LOOP ( 'NONE', ( #13505, #9026, #10268, #1632 ) ) ;
#10945=DIRECTION ( 'NONE',  ( 0.000000000000000000, 1.000000000000000000, 0.000000000000000000 ) ) ;
#10951=ORIENTED_EDGE ( 'NONE', *, *, #3046, .T. ) ;
#10956=ADVANCED_FACE ( 'NONE', ( #7306 ), #10273, .T. ) ;
#10957=DIRECTION ( 'NONE',  ( 0.000000000000000000, 0.000000000000000000, 1.000000000000000000 ) ) ;
#10960=ADVANCED_FACE ( 'NONE', ( #3995 ), #12689, .T. ) ;
#10963=CARTESIAN_POINT ( 'NONE',  ( -11.46847481510586775, 0.000000000000000000, -5.708888906988912382 ) ) ;
#10964=CARTESIAN_POINT ( 'NONE',  ( -2.161962830978702677, 0.000000000000000000, 14.08504230442587435 ) ) ;
#10967=ORIENTED_EDGE ( 'NONE', *, *, #8053, .F. ) ;
#10972=CARTESIAN_POINT ( 'NONE',  ( 12.03251085770905959, 3.000000000000000000, 3.999999998926332179 ) ) ;
#10974=CARTESIAN_POINT ( 'NONE',  ( -8.771102293099080072, 0.000000000000000000, -10.33484986938307770 ) ) ;
#10981=ORIENTED_EDGE ( 'NONE', *, *, #13300, .F. ) ;
#10992=AXIS2_PLACEMENT_3D ( 'NONE', #10349, #2021, #10288 ) ;
#11002=CIRCLE ( 'NONE', #5068, 14.25000000000000178 ) ;
#11004=B_SPLINE_CURVE_WITH_KNOTS ( 'NONE', 3,
 ( #755, #8993, #8111, #1925 ),
 .UNSPECIFIED., .F., .F.,
 ( 4, 4 ),
 ( 0.000000000000000000, 0.8452273900860258760 ),
 .UNSPECIFIED. ) ;
#11010=CIRCLE ( 'NONE', #40, 14.25000000000000178 ) ;
#11011=CARTESIAN_POINT ( 'NONE',  ( 0.000000000000000000, 3.000000000000000000, 0.000000000000000000 ) ) ;
#11017=EDGE_CURVE ( 'NONE', #3089, #655, #2265, .T. ) ;
#11018=ORIENTED_EDGE ( 'NONE', *, *, #2072, .T. ) ;
#11025=CARTESIAN_POINT ( 'NONE',  ( 0.7901945867173618687, 3.000000000000000000, 12.78643498603817541 ) ) ;
#11026=CARTESIAN_POINT ( 'NONE',  ( 13.04554897075799502, 3.000000000000000000, 5.733772933379473358 ) ) ;
#11029=ORIENTED_EDGE ( 'NONE', *, *, #2874, .F. ) ;
#11036=ORIENTED_EDGE ( 'NONE', *, *, #8687, .F. ) ;
#11037=EDGE_CURVE ( 'NONE', #6668, #5900, #9052, .T. ) ;
#11038=EDGE_CURVE ( 'NONE', #3932, #1933, #5299, .T. ) ;
#11044=DIRECTION ( 'NONE',  ( 0.000000000000000000, 0.000000000000000000, -1.000000000000000000 ) ) ;
#11046=DIRECTION ( 'NONE',  ( -0.000000000000000000, -1.000000000000000000, -0.000000000000000000 ) ) ;
#11049=CARTESIAN_POINT ( 'NONE',  ( 10.67828022838850366, 3.000000000000000000, -7.077546079049271022 ) ) ;
#11050=DIRECTION ( 'NONE',  ( -1.000000000000000000, 0.000000000000000000, 9.145772869372436484E-17 ) ) ;
#11055=VECTOR ( 'NONE', #10433, 1000.000000000000000 ) ;
#11056=PRODUCT_DEFINITION_SHAPE ( 'NONE', 'NONE',  #5706 ) ;
#11058=ORIENTED_EDGE ( 'NONE', *, *, #986, .T. ) ;
#11069=EDGE_CURVE ( 'NONE', #843, #4282, #10434, .T. ) ;
#11076=CIRCLE ( 'NONE', #9967, 12.08999999999737440 ) ;
#11089=ORIENTED_EDGE ( 'NONE', *, *, #8394, .F. ) ;
#11091=ORIENTED_EDGE ( 'NONE', *, *, #7823, .T. ) ;
#11096=CARTESIAN_POINT ( 'NONE',  ( -11.14709020439930676, 0.000000000000000000, -7.712570079660886257 ) ) ;
#11105=CARTESIAN_POINT ( 'NONE',  ( 8.482622935103764306, 3.000000000000000000, -9.600126836553261711 ) ) ;
#11106=CARTESIAN_POINT ( 'NONE',  ( -1.119409668803374558, 0.000000000000000000, -13.50845331674225669 ) ) ;
#11112=ORIENTED_EDGE ( 'NONE', *, *, #6422, .T. ) ;
#11113=CYLINDRICAL_SURFACE ( 'NONE', #4235, 12.08999999999737440 ) ;
#11117=CARTESIAN_POINT ( 'NONE',  ( 8.922226997226882617, 3.000000000000000000, 8.158551673544282679 ) ) ;
#11118=CARTESIAN_POINT ( 'NONE',  ( -8.914835885878284572, 3.000000000000000000, -11.11702303352191379 ) ) ;
#11119=DIRECTION ( 'NONE',  ( 0.000000000000000000, 1.000000000000000000, 0.000000000000000000 ) ) ;
#11120=EDGE_CURVE ( 'NONE', #4282, #843, #3597, .T. ) ;
#11122=CARTESIAN_POINT ( 'NONE',  ( -5.170206418547117266, 3.000000000000000000, 13.27898586450088203 ) ) ;
#11126=CARTESIAN_POINT ( 'NONE',  ( -14.08504230442586369, 0.000000000000000000, 2.161962830978781724 ) ) ;
#11127=CARTESIAN_POINT ( 'NONE',  ( 5.571313494980132397, 3.000000000000000000, -10.72979803820131472 ) ) ;
#11134=ORIENTED_EDGE ( 'NONE', *, *, #5581, .F. ) ;
#11137=CARTESIAN_POINT ( 'NONE',  ( -11.11702303352197063, 0.000000000000000000, -8.914835885878215294 ) ) ;
#11143=ORIENTED_EDGE ( 'NONE', *, *, #8101, .T. ) ;
#11145=VERTEX_POINT ( 'NONE', #619 ) ;
#11147=EDGE_LOOP ( 'NONE', ( #6535, #12740, #13262, #1451 ) ) ;
#11149=CARTESIAN_POINT ( 'NONE',  ( 10.72979803820131472, 0.000000000000000000, 5.571313494980131509 ) ) ;
#11151=CARTESIAN_POINT ( 'NONE',  ( 1.557181465540758758, 3.000000000000000000, 14.16466328168009881 ) ) ;
#11154=CARTESIAN_POINT ( 'NONE',  ( 0.000000000000000000, 3.000000000000000000, 0.000000000000000000 ) ) ;
#11156=ORIENTED_EDGE ( 'NONE', *, *, #3046, .F. ) ;
#11157=CARTESIAN_POINT ( 'NONE',  ( -5.731782959214987372, 0.000000000000000000, -11.46814821560793618 ) ) ;
#11161=ORIENTED_EDGE ( 'NONE', *, *, #10779, .F. ) ;
#11170=CARTESIAN_POINT ( 'NONE',  ( -6.506507307819711095, 3.000000000000000000, 10.18987059060247624 ) ) ;
#11172=ORIENTED_EDGE ( 'NONE', *, *, #7671, .F. ) ;
#11173=CARTESIAN_POINT ( 'NONE',  ( 0.000000000000000000, 3.000000000000000000, 0.000000000000000000 ) ) ;
#11174=ORIENTED_EDGE ( 'NONE', *, *, #12015, .T. ) ;
#11175=B_SPLINE_CURVE_WITH_KNOTS ( 'NONE', 3,
 ( #9994, #10963, #495, #3793 ),
 .UNSPECIFIED., .F., .F.,
 ( 4, 4 ),
 ( 0.1547128134717859205, 1.000000000000000000 ),
 .UNSPECIFIED. ) ;
#11197=CARTESIAN_POINT ( 'NONE',  ( -8.760376775873710997, 0.000000000000000000, 10.34346111134700941 ) ) ;
#11205=ORIENTED_EDGE ( 'NONE', *, *, #3314, .F. ) ;
#11213=CARTESIAN_POINT ( 'NONE',  ( -8.430890348300632553, 0.000000000000000000, -11.48836750521723538 ) ) ;
#11218=CARTESIAN_POINT ( 'NONE',  ( -3.647470871583628593, 3.000000000000000000, 11.52666717836884125 ) ) ;
#11221=CARTESIAN_POINT ( 'NONE',  ( -13.27898586450070084, 3.000000000000000000, -5.170206418547588001 ) ) ;
#11223=EDGE_CURVE ( 'NONE', #7786, #3089, #8724, .T. ) ;
#11224=ORIENTED_EDGE ( 'NONE', *, *, #11243, .T. ) ;
#11226=ORIENTED_EDGE ( 'NONE', *, *, #6184, .F. ) ;
#11229=DIRECTION ( 'NONE',  ( 0.000000000000000000, 0.000000000000000000, -1.000000000000000000 ) ) ;
#11230=EDGE_CURVE ( 'NONE', #9838, #1063, #2084, .T. ) ;
#11234=VECTOR ( 'NONE', #5894, 1000.000000000000000 ) ;
#11238=CARTESIAN_POINT ( 'NONE',  ( -13.50845331674225847, 0.000000000000000000, 1.119409668803372115 ) ) ;
#11243=EDGE_CURVE ( 'NONE', #1347, #911, #2749, .T. ) ;
#11245=ADVANCED_FACE ( 'NONE', ( #3698, #8999, #3568 ), #13214, .F. ) ;
#11252=CARTESIAN_POINT ( 'NONE',  ( -13.33788847341978645, 3.000000000000000000, -2.414978278956336322 ) ) ;
#11253=CARTESIAN_POINT ( 'NONE',  ( -8.504652361247167391, 0.000000000000000000, -9.593885948927674434 ) ) ;
#11259=LINE ( 'NONE', #7872, #9040 ) ;
#11261=CARTESIAN_POINT ( 'NONE',  ( -4.577511697546077230, 3.000000000000000000, -12.75843939030334795 ) ) ;
#11264=VERTEX_POINT ( 'NONE', #13087 ) ;
#11266=ORIENTED_EDGE ( 'NONE', *, *, #8394, .T. ) ;
#11277=CARTESIAN_POINT ( 'NONE',  ( -12.07794044664754018, 0.000000000000000000, -0.5398653231797256868 ) ) ;
#11285=CIRCLE ( 'NONE', #7114, 14.25000000000000178 ) ;
#11290=CARTESIAN_POINT ( 'NONE',  ( 8.430890348300586368, 3.000000000000000000, -11.48836750521726913 ) ) ;
#11294=DIRECTION ( 'NONE',  ( 0.000000000000000000, 1.000000000000000000, 0.000000000000000000 ) ) ;
#11304=VERTEX_POINT ( 'NONE', #9213 ) ;
#11306=ORIENTED_EDGE ( 'NONE', *, *, #2071, .T. ) ;
#11314=LINE ( 'NONE', #11513, #10378 ) ;
#11315=CARTESIAN_POINT ( 'NONE',  ( -11.46847481510586775, 3.000000000000000000, -5.708888906988912382 ) ) ;
#11321=VERTEX_POINT ( 'NONE', #11425 ) ;
#11323=CARTESIAN_POINT ( 'NONE',  ( -0.5398653231797316820, 3.000000000000000000, 12.07794044664754018 ) ) ;
#11328=DIRECTION ( 'NONE',  ( 0.000000000000000000, 1.000000000000000000, 0.000000000000000000 ) ) ;
#11332=CARTESIAN_POINT ( 'NONE',  ( 1.557181465540758758, 3.000000000000000000, 14.16466328168009881 ) ) ;
#11335=LINE ( 'NONE', #8218, #6852 ) ;
#11336=CARTESIAN_POINT ( 'NONE',  ( 13.27898586450067420, 3.000000000000000000, 5.170206418547648397 ) ) ;
#11337=FACE_OUTER_BOUND ( 'NONE', #9796, .T. ) ;
#11342=ORIENTED_EDGE ( 'NONE', *, *, #6420, .F. ) ;
#11343=LINE ( 'NONE', #8356, #13500 ) ;
#11344=CARTESIAN_POINT ( 'NONE',  ( 0.000000000000000000, 0.000000000000000000, 0.000000000000000000 ) ) ;
#11348=CYLINDRICAL_SURFACE ( 'NONE', #7295, 12.08999999999737440 ) ;
#11362=CARTESIAN_POINT ( 'NONE',  ( 1.105736515254441388, 0.000000000000000000, -13.50994833511691695 ) ) ;
#11363=CARTESIAN_POINT ( 'NONE',  ( 11.48836750521724070, 3.000000000000000000, 8.430890348300627224 ) ) ;
#11373=ORIENTED_EDGE ( 'NONE', *, *, #2072, .F. ) ;
#11383=CARTESIAN_POINT ( 'NONE',  ( -11.52666717836884125, 3.000000000000000000, -3.647470871583627705 ) ) ;
#11385=B_SPLINE_CURVE_WITH_KNOTS ( 'NONE', 3,
 ( #4792, #6854, #1764, #8978 ),
 .UNSPECIFIED., .F., .F.,
 ( 4, 4 ),
 ( 0.000000000000000000, 0.8452273900860258760 ),
 .UNSPECIFIED. ) ;
#11386=ADVANCED_FACE ( 'NONE', ( #12482 ), #387, .F. ) ;
#11387=ORIENTED_EDGE ( 'NONE', *, *, #6021, .T. ) ;
#11389=FACE_OUTER_BOUND ( 'NONE', #4740, .T. ) ;
#11390=EDGE_CURVE ( 'NONE', #5917, #13298, #5110, .T. ) ;
#11393=CARTESIAN_POINT ( 'NONE',  ( 3.647599401157688437, 0.000000000000000000, 11.52662650599083882 ) ) ;
#11404=EDGE_CURVE ( 'NONE', #5785, #9584, #327, .T. ) ;
#11408=DIRECTION ( 'NONE',  ( 0.000000000000000000, 0.000000000000000000, 1.000000000000000000 ) ) ;
#11409=EDGE_CURVE ( 'NONE', #7235, #10517, #12337, .T. ) ;
#11413=FACE_OUTER_BOUND ( 'NONE', #5423, .T. ) ;
#11414=DIRECTION ( 'NONE',  ( 0.000000000000000000, 0.000000000000000000, 1.000000000000000000 ) ) ;
#11416=CARTESIAN_POINT ( 'NONE',  ( 0.000000000000000000, 3.000000000000000000, 0.000000000000000000 ) ) ;
#11417=EDGE_CURVE ( 'NONE', #3822, #9443, #6933, .T. ) ;
#11421=DIRECTION ( 'NONE',  ( 0.000000000000000000, 0.000000000000000000, -1.000000000000000000 ) ) ;
#11423=DIRECTION ( 'NONE',  ( 0.000000000000000000, 1.000000000000000000, 0.000000000000000000 ) ) ;
#11425=CARTESIAN_POINT ( 'NONE',  ( 2.604399508763944660, 0.000000000000000000, -11.80615107470197600 ) ) ;
#11432=VERTEX_POINT ( 'NONE', #11831 ) ;
#11434=DIRECTION ( 'NONE',  ( 0.000000000000000000, 0.000000000000000000, -1.000000000000000000 ) ) ;
#11440=DIRECTION ( 'NONE',  ( -0.000000000000000000, -1.000000000000000000, -0.000000000000000000 ) ) ;
#11443=DIRECTION ( 'NONE',  ( 0.000000000000000000, 0.000000000000000000, 1.000000000000000000 ) ) ;
#11444=ORIENTED_EDGE ( 'NONE', *, *, #4337, .F. ) ;
#11448=AXIS2_PLACEMENT_3D ( 'NONE', #7524, #7835, #12764 ) ;
#11449=CIRCLE ( 'NONE', #2429, 14.25000000000000355 ) ;
#11452=CARTESIAN_POINT ( 'NONE',  ( -5.731782959214987372, 0.000000000000000000, -11.46814821560793618 ) ) ;
#11459=EDGE_CURVE ( 'NONE', #3932, #9838, #2639, .T. ) ;
#11462=CIRCLE ( 'NONE', #9029, 12.08999999999737263 ) ;
#11468=ORIENTED_EDGE ( 'NONE', *, *, #7913, .F. ) ;
#11471=DIRECTION ( 'NONE',  ( 0.000000000000000000, 0.000000000000000000, 1.000000000000000000 ) ) ;
#11473=CIRCLE ( 'NONE', #3283, 4.000000000000000000 ) ;
#11476=CARTESIAN_POINT ( 'NONE',  ( 0.5398653231797245766, 3.000000000000000000, -12.07794044664754018 ) ) ;
#11477=CARTESIAN_POINT ( 'NONE',  ( 1.557181465540758758, 3.000000000000000000, 14.16466328168009881 ) ) ;
#11482=CARTESIAN_POINT ( 'NONE',  ( 13.04554897075799502, 0.000000000000000000, 5.733772933379473358 ) ) ;
#11491=CARTESIAN_POINT ( 'NONE',  ( 5.170206418547604876, 0.000000000000000000, -13.27898586450069196 ) ) ;
#11495=CARTESIAN_POINT ( 'NONE',  ( -11.11702303352197063, 0.000000000000000000, -8.914835885878215294 ) ) ;
#11501=AXIS2_PLACEMENT_3D ( 'NONE', #3939, #10348, #13460 ) ;
#11504=DIRECTION ( 'NONE',  ( 0.000000000000000000, 0.000000000000000000, 1.000000000000000000 ) ) ;
#11505=( NAMED_UNIT ( * ) PLANE_ANGLE_UNIT ( ) SI_UNIT ( $, .RADIAN. ) );
#11506=CARTESIAN_POINT ( 'NONE',  ( -8.430890348300124515, 0.000000000000000000, 11.48836750521761019 ) ) ;
#11507=DIRECTION ( 'NONE',  ( 0.000000000000000000, 0.000000000000000000, -1.000000000000000000 ) ) ;
#11512=STYLED_ITEM('',(#13642),#8440);
#11513=CARTESIAN_POINT ( 'NONE',  ( 6.506620931068707314, 3.000000000000000000, 10.18979803820051622 ) ) ;
#11514=CARTESIAN_POINT ( 'NONE',  ( -11.46847481510586775, 0.000000000000000000, -5.708888906988912382 ) ) ;
#11518=ORIENTED_EDGE ( 'NONE', *, *, #987, .T. ) ;
#11526=CARTESIAN_POINT ( 'NONE',  ( 0.5398653231797245766, 3.000000000000000000, -12.07794044664754018 ) ) ;
#11528=CARTESIAN_POINT ( 'NONE',  ( -5.784789447945489549, 3.000000000000000000, 12.25836857253663581 ) ) ;
#11533=ORIENTED_EDGE ( 'NONE', *, *, #8254, .T. ) ;
#11537=VERTEX_POINT ( 'NONE', #5553 ) ;
#11543=DIRECTION ( 'NONE',  ( -0.000000000000000000, -1.000000000000000000, -0.000000000000000000 ) ) ;
#11547=EDGE_CURVE ( 'NONE', #10838, #1061, #7787, .T. ) ;
#11549=AXIS2_PLACEMENT_3D ( 'NONE', #2087, #6348, #10493 ) ;
#11550=DIRECTION ( 'NONE',  ( -0.000000000000000000, -1.000000000000000000, -0.000000000000000000 ) ) ;
#11553=B_SPLINE_CURVE_WITH_KNOTS ( 'NONE', 3,
 ( #10497, #9394, #798, #5118 ),
 .UNSPECIFIED., .F., .F.,
 ( 4, 4 ),
 ( 0.1547128134717859205, 1.000000000000000000 ),
 .UNSPECIFIED. ) ;
#11556=VECTOR ( 'NONE', #10760, 1000.000000000000000 ) ;
#11558=CARTESIAN_POINT ( 'NONE',  ( 31.00000000000000000, 0.000000000000000000, -4.000000001073670930 ) ) ;
#11561=EDGE_CURVE ( 'NONE', #2665, #10780, #10228, .T. ) ;
#11564=FACE_OUTER_BOUND ( 'NONE', #946, .T. ) ;
#11571=CARTESIAN_POINT ( 'NONE',  ( 3.647470871583629926, 0.000000000000000000, -11.52666717836884125 ) ) ;
#11576=ORIENTED_EDGE ( 'NONE', *, *, #13410, .F. ) ;
#11578=LINE ( 'NONE', #2131, #2701 ) ;
#11582=CARTESIAN_POINT ( 'NONE',  ( -13.27898586450066709, 0.000000000000000000, 5.170206418547661720 ) ) ;
#11583=CARTESIAN_POINT ( 'NONE',  ( -11.11702303352197063, 3.000000000000000000, -8.914835885878215294 ) ) ;
#11589=VERTEX_POINT ( 'NONE', #4797 ) ;
#11593=ADVANCED_FACE ( 'NONE', ( #3482 ), #10094, .T. ) ;
#11600=CARTESIAN_POINT ( 'NONE',  ( -2.546103534247749600, 3.000000000000000000, 12.55526518755974585 ) ) ;
#11603=CARTESIAN_POINT ( 'NONE',  ( 31.00000000000000000, 3.000000000000000000, -4.000000001073670930 ) ) ;
#11605=CARTESIAN_POINT ( 'NONE',  ( 11.46814821560793618, 3.000000000000000000, -5.731782959214992701 ) ) ;
#11606=B_SPLINE_SURFACE_WITH_KNOTS ( 'NONE', 3, 1, ( 
 ( #10582, #6304 ),
 ( #55, #1789 ),
 ( #12718, #7476 ),
 ( #11218, #2111 ) ),
 .UNSPECIFIED., .F., .F., .F.,
 ( 4, 4 ),
 ( 2, 2 ),
 ( 0.000000000000000000, 0.8452273900860258760 ),
 ( 0.000000000000000000, 1.000000000000000000 ),
 .UNSPECIFIED. ) ;
#11609=ORIENTED_EDGE ( 'NONE', *, *, #9016, .T. ) ;
#11617=ADVANCED_FACE ( 'NONE', ( #2730 ), #5541, .F. ) ;
#11620=B_SPLINE_SURFACE_WITH_KNOTS ( 'NONE', 3, 1, ( 
 ( #5083, #2747 ),
 ( #2951, #11362 ),
 ( #1988, #823 ),
 ( #6121, #958 ) ),
 .UNSPECIFIED., .F., .F., .F.,
 ( 4, 4 ),
 ( 2, 2 ),
 ( 0.000000000000000000, 0.8452273900860258760 ),
 ( 0.000000000000000000, 1.000000000000000000 ),
 .UNSPECIFIED. ) ;
#11622=ORIENTED_EDGE ( 'NONE', *, *, #12061, .F. ) ;
#11624=CARTESIAN_POINT ( 'NONE',  ( 0.000000000000000000, 3.000000000000000000, 0.000000000000000000 ) ) ;
#11626=FACE_OUTER_BOUND ( 'NONE', #6865, .T. ) ;
#11628=CARTESIAN_POINT ( 'NONE',  ( -11.46847481510586775, 3.000000000000000000, -5.708888906988912382 ) ) ;
#11636=ORIENTED_EDGE ( 'NONE', *, *, #4378, .T. ) ;
#11640=CARTESIAN_POINT ( 'NONE',  ( 0.000000000000000000, 3.000000000000000000, 0.000000000000000000 ) ) ;
#11641=CARTESIAN_POINT ( 'NONE',  ( 5.708888906988906164, 3.000000000000000000, -11.46847481510586775 ) ) ;
#11642=CARTESIAN_POINT ( 'NONE',  ( 0.000000000000000000, 0.000000000000000000, 0.000000000000000000 ) ) ;
#11643=CYLINDRICAL_SURFACE ( 'NONE', #6818, 14.25000000000000000 ) ;
#11645=CARTESIAN_POINT ( 'NONE',  ( 8.922136023539611216, 0.000000000000000000, -8.158651161643899030 ) ) ;
#11650=VECTOR ( 'NONE', #7699, 1000.000000000000000 ) ;
#11655=CARTESIAN_POINT ( 'NONE',  ( -12.55526518755974585, 0.000000000000000000, -2.546103534247746047 ) ) ;
#11657=CARTESIAN_POINT ( 'NONE',  ( 31.00000000000000000, 0.000000000000000000, -1.500000000759764029 ) ) ;
#11659=CARTESIAN_POINT ( 'NONE',  ( -12.76342233970728124, 0.000000000000000000, -4.564691384634500970 ) ) ;
#11661=EDGE_CURVE ( 'NONE', #1061, #3195, #8898, .T. ) ;
#11662=CARTESIAN_POINT ( 'NONE',  ( 0.000000000000000000, 3.000000000000000000, 0.000000000000000000 ) ) ;
#11667=ORIENTED_EDGE ( 'NONE', *, *, #2447, .F. ) ;
#11671=ORIENTED_EDGE ( 'NONE', *, *, #5862, .T. ) ;
#11672=DIRECTION ( 'NONE',  ( 0.000000000000000000, 1.000000000000000000, 0.000000000000000000 ) ) ;
#11675=VECTOR ( 'NONE', #6122, 1000.000000000000000 ) ;
#11680=VERTEX_POINT ( 'NONE', #12640 ) ;
#11683=AXIS2_PLACEMENT_3D ( 'NONE', #9610, #186, #9810 ) ;
#11688=EDGE_CURVE ( 'NONE', #1091, #5675, #12515, .T. ) ;
#11689=CARTESIAN_POINT ( 'NONE',  ( 31.00000000000000000, 3.000000000000000000, -1.073670993220974656E-09 ) ) ;
#11691=CARTESIAN_POINT ( 'NONE',  ( 2.604531154829233586, 3.000000000000000000, 11.80612203322752585 ) ) ;
#11694=CARTESIAN_POINT ( 'NONE',  ( 3.647599401157691101, 3.000000000000000000, 11.52662650599084238 ) ) ;
#11698=ORIENTED_EDGE ( 'NONE', *, *, #4536, .F. ) ;
#11699=CARTESIAN_POINT ( 'NONE',  ( -2.161962830978783057, 3.000000000000000000, -14.08504230442586369 ) ) ;
#11701=AXIS2_PLACEMENT_3D ( 'NONE', #11011, #9977, #9903 ) ;
#11704=DIRECTION ( 'NONE',  ( 0.000000000000000000, 0.000000000000000000, 1.000000000000000000 ) ) ;
#11705=B_SPLINE_SURFACE_WITH_KNOTS ( 'NONE', 3, 1, ( 
 ( #10167, #13552 ),
 ( #4107, #744 ),
 ( #1846, #5006 ),
 ( #9139, #11277 ) ),
 .UNSPECIFIED., .F., .F., .F.,
 ( 4, 4 ),
 ( 2, 2 ),
 ( 0.000000000000000000, 0.8452273900860258760 ),
 ( 0.000000000000000000, 1.000000000000000000 ),
 .UNSPECIFIED. ) ;
#11707=CARTESIAN_POINT ( 'NONE',  ( 0.000000000000000000, 3.000000000000000000, 0.000000000000000000 ) ) ;
#11714=CARTESIAN_POINT ( 'NONE',  ( -11.11702303352197063, 3.000000000000000000, -8.914835885878215294 ) ) ;
#11718=VERTEX_POINT ( 'NONE', #7262 ) ;
#11719=ORIENTED_EDGE ( 'NONE', *, *, #5835, .T. ) ;
#11720=CARTESIAN_POINT ( 'NONE',  ( 5.571313494980132397, 0.000000000000000000, -10.72979803820131472 ) ) ;
#11725=CIRCLE ( 'NONE', #3353, 12.08999999999737440 ) ;
#11728=AXIS2_PLACEMENT_3D ( 'NONE', #2478, #3371, #3499 ) ;
#11731=FACE_BOUND ( 'NONE', #4079, .T. ) ;
#11738=CARTESIAN_POINT ( 'NONE',  ( -13.27898586450066709, 0.000000000000000000, 5.170206418547661720 ) ) ;
#11753=ORIENTED_EDGE ( 'NONE', *, *, #531, .T. ) ;
#11754=ORIENTED_EDGE ( 'NONE', *, *, #8881, .F. ) ;
#11756=VECTOR ( 'NONE', #875, 1000.000000000000000 ) ;
#11759=ORIENTED_EDGE ( 'NONE', *, *, #2554, .F. ) ;
#11769=CARTESIAN_POINT ( 'NONE',  ( 0.7702044561450380744, 0.000000000000000000, -12.79759916868914615 ) ) ;
#11770=EDGE_LOOP ( 'NONE', ( #8941, #3373, #5600, #947, #5025, #806, #8371, #4764, #12736, #9310, #3949, #10533, #7535, #11997, #8533, #3858, #4518, #12898, #13090, #4563, #10933, #8118, #7827, #6692, #3661, #3177, #8583, #4960, #7041, #4123, #10723, #9859, #2788, #10173, #1931, #6869, #6503, #6155, #1572, #3434, #10234, #6995, #8200, #6945, #10657, #1717, #12641, #8203, #401, #11533, #10054, #7387, #2856, #7678, #12713, #8042, #9800, #12678, #149, #12970, #12382, #4414, #7908, #410, #7283, #5563, #11018, #10692, #3616, #11609, #7565, #8989, #4008, #5574, #7313, #13055, #9411, #11671, #163, #8977, #399, #1487, #5410, #8620, #340, #11849, #2719, #11058, #11387, #3452, #9455 ) ) ;
#11773=DIRECTION ( 'NONE',  ( 0.000000000000000000, 1.000000000000000000, 0.000000000000000000 ) ) ;
#11781=CARTESIAN_POINT ( 'NONE',  ( 0.000000000000000000, 3.000000000000000000, 0.000000000000000000 ) ) ;
#11785=CARTESIAN_POINT ( 'NONE',  ( -14.16466328168010769, 3.000000000000000000, -1.557181465540673271 ) ) ;
#11788=EDGE_CURVE ( 'NONE', #1501, #6519, #3288, .T. ) ;
#11794=CARTESIAN_POINT ( 'NONE',  ( 13.27898586450067242, 3.000000000000000000, -5.170206418547655502 ) ) ;
#11799=CARTESIAN_POINT ( 'NONE',  ( 2.161962830978694683, 3.000000000000000000, -14.08504230442587790 ) ) ;
#11807=VERTEX_POINT ( 'NONE', #1126 ) ;
#11808=EDGE_CURVE ( 'NONE', #10780, #2104, #8245, .T. ) ;
#11811=ADVANCED_FACE ( 'NONE', ( #8346 ), #3115, .F. ) ;
#11818=DIRECTION ( 'NONE',  ( 0.000000000000000000, 0.000000000000000000, 1.000000000000000000 ) ) ;
#11822=CARTESIAN_POINT ( 'NONE',  ( 8.922226997226887946, 0.000000000000000000, 8.158551673544288008 ) ) ;
#11825=ORIENTED_EDGE ( 'NONE', *, *, #13564, .T. ) ;
#11826=CARTESIAN_POINT ( 'NONE',  ( -8.914835885878215294, 3.000000000000000000, 11.11702303352197063 ) ) ;
#11831=CARTESIAN_POINT ( 'NONE',  ( 13.27898586450067420, 0.000000000000000000, 5.170206418547648397 ) ) ;
#11834=ADVANCED_FACE ( 'NONE', ( #3451 ), #174, .T. ) ;
#11835=CARTESIAN_POINT ( 'NONE',  ( 8.158651161643900807, 3.000000000000000000, 8.922136023539609440 ) ) ;
#11839=VERTEX_POINT ( 'NONE', #10964 ) ;
#11848=CARTESIAN_POINT ( 'NONE',  ( 0.000000000000000000, 3.000000000000000000, 0.000000000000000000 ) ) ;
#11849=ORIENTED_EDGE ( 'NONE', *, *, #5007, .T. ) ;
#11851=VERTEX_POINT ( 'NONE', #8614 ) ;
#11855=ORIENTED_EDGE ( 'NONE', *, *, #9212, .F. ) ;
#11865=ORIENTED_EDGE ( 'NONE', *, *, #13578, .T. ) ;
#11868=ORIENTED_EDGE ( 'NONE', *, *, #11404, .F. ) ;
#11870=AXIS2_PLACEMENT_3D ( 'NONE', #13359, #8046, #4871 ) ;
#11874=EDGE_CURVE ( 'NONE', #4083, #10517, #550, .T. ) ;
#11878=CARTESIAN_POINT ( 'NONE',  ( -12.07794044664754018, 0.000000000000000000, -0.5398653231797256868 ) ) ;
#11880=CIRCLE ( 'NONE', #5065, 14.24999999999999822 ) ;
#11889=EDGE_CURVE ( 'NONE', #10564, #5245, #6561, .T. ) ;
#11891=AXIS2_PLACEMENT_3D ( 'NONE', #3362, #12744, #11507 ) ;
#11893=LINE ( 'NONE', #1563, #5510 ) ;
#11894=DIRECTION ( 'NONE',  ( 0.000000000000000000, 1.000000000000000000, 0.000000000000000000 ) ) ;
#11900=ORIENTED_EDGE ( 'NONE', *, *, #7541, .F. ) ;
#11902=ORIENTED_EDGE ( 'NONE', *, *, #5070, .T. ) ;
#11906=CARTESIAN_POINT ( 'NONE',  ( -2.428572470324203980, 3.000000000000000000, -13.33579367773357482 ) ) ;
#11907=VERTEX_POINT ( 'NONE', #12767 ) ;
#11909=EDGE_CURVE ( 'NONE', #116, #6616, #7528, .T. ) ;
#11913=DIRECTION ( 'NONE',  ( 0.000000000000000000, 1.000000000000000000, 0.000000000000000000 ) ) ;
#11915=FACE_OUTER_BOUND ( 'NONE', #4364, .T. ) ;
#11920=PRODUCT_DEFINITION_CONTEXT ( 'detailed design', #2041, 'design' ) ;
#11922=CARTESIAN_POINT ( 'NONE',  ( 5.733772933379474246, 0.000000000000000000, -13.04554897075799502 ) ) ;
#11930=CARTESIAN_POINT ( 'NONE',  ( 2.414978278956333213, 3.000000000000000000, -13.33788847341978645 ) ) ;
#11934=AXIS2_PLACEMENT_3D ( 'NONE', #4514, #3332, #11818 ) ;
#11938=ORIENTED_EDGE ( 'NONE', *, *, #9649, .T. ) ;
#11941=VERTEX_POINT ( 'NONE', #496 ) ;
#11946=AXIS2_PLACEMENT_3D ( 'NONE', #1963, #4096, #3054 ) ;
#11949=CARTESIAN_POINT ( 'NONE',  ( 3.647470871583629926, 3.000000000000000000, -11.52666717836884125 ) ) ;
#11950=CARTESIAN_POINT ( 'NONE',  ( 10.69794375946289655, 0.000000000000000000, 7.065816209474157006 ) ) ;
#11962=CARTESIAN_POINT ( 'NONE',  ( -8.482622935103766082, 3.000000000000000000, 9.600126836553263487 ) ) ;
#11966=CARTESIAN_POINT ( 'NONE',  ( 8.430890348300625448, 3.000000000000000000, 11.48836750521723893 ) ) ;
#11970=CARTESIAN_POINT ( 'NONE',  ( 13.27898586450067242, 0.000000000000000000, -5.170206418547655502 ) ) ;
#11971=CARTESIAN_POINT ( 'NONE',  ( 0.000000000000000000, 3.000000000000000000, 0.000000000000000000 ) ) ;
#11977=ORIENTED_EDGE ( 'NONE', *, *, #11547, .F. ) ;
#11978=ADVANCED_FACE ( 'NONE', ( #5718 ), #1607, .F. ) ;
#11983=ORIENTED_EDGE ( 'NONE', *, *, #1701, .F. ) ;
#11993=DIRECTION ( 'NONE',  ( -0.000000000000000000, -1.000000000000000000, -0.000000000000000000 ) ) ;
#11997=ORIENTED_EDGE ( 'NONE', *, *, #11459, .T. ) ;
#12002=EDGE_LOOP ( 'NONE', ( #3027, #3133 ) ) ;
#12007=CARTESIAN_POINT ( 'NONE',  ( 31.00000000000000000, 3.000000000000000000, -1.073670993220974656E-09 ) ) ;
#12015=EDGE_CURVE ( 'NONE', #7310, #11432, #8026, .T. ) ;
#12018=B_SPLINE_CURVE_WITH_KNOTS ( 'NONE', 3,
 ( #5830, #1707, #6858, #8982 ),
 .UNSPECIFIED., .F., .F.,
 ( 4, 4 ),
 ( 0.000000000000000000, 0.8452273900860258760 ),
 .UNSPECIFIED. ) ;
#12023=CARTESIAN_POINT ( 'NONE',  ( 12.48034623170854474, 3.000000000000000000, 4.337627373772809491 ) ) ;
#12030=CARTESIAN_POINT ( 'NONE',  ( 5.571433138827823761, 3.000000000000000000, 10.72973591378220704 ) ) ;
#12031=CARTESIAN_POINT ( 'NONE',  ( -13.50994833511691340, 0.000000000000000000, -1.105736515254444052 ) ) ;
#12039=LINE ( 'NONE', #3755, #1779 ) ;
#12040=EDGE_CURVE ( 'NONE', #8456, #4963, #3190, .T. ) ;
#12046=VERTEX_POINT ( 'NONE', #9022 ) ;
#12060=CARTESIAN_POINT ( 'NONE',  ( -5.731782959214987372, 3.000000000000000000, -11.46814821560793618 ) ) ;
#12061=EDGE_CURVE ( 'NONE', #11907, #9840, #3847, .T. ) ;
#12063=UNCERTAINTY_MEASURE_WITH_UNIT (LENGTH_MEASURE( 1.000000000000000082E-05 ), #8067, 'distance_accuracy_value', 'NONE');
#12067=VERTEX_POINT ( 'NONE', #1943 ) ;
#12071=EDGE_CURVE ( 'NONE', #6591, #1437, #1490, .T. ) ;
#12077=LINE ( 'NONE', #783, #286 ) ;
#12084=DIRECTION ( 'NONE',  ( -0.000000000000000000, -1.000000000000000000, -0.000000000000000000 ) ) ;
#12091=CARTESIAN_POINT ( 'NONE',  ( -8.430890348300632553, 0.000000000000000000, -11.48836750521723538 ) ) ;
#12094=CARTESIAN_POINT ( 'NONE',  ( 0.5400000000008001733, 3.000000000000000000, 12.07793442604883616 ) ) ;
#12099=FACE_OUTER_BOUND ( 'NONE', #4610, .T. ) ;
#12100=CARTESIAN_POINT ( 'NONE',  ( 6.506620931068707314, 0.000000000000000000, 10.18979803820051622 ) ) ;
#12101=EDGE_CURVE ( 'NONE', #284, #4963, #91, .T. ) ;
#12102=CARTESIAN_POINT ( 'NONE',  ( 0.000000000000000000, 0.000000000000000000, 0.000000000000000000 ) ) ;
#12107=CARTESIAN_POINT ( 'NONE',  ( 12.01285915242476499, 3.000000000000000000, -4.000000001073668265 ) ) ;
#12108=CARTESIAN_POINT ( 'NONE',  ( -11.48836750521728689, 0.000000000000000000, -8.430890348300561499 ) ) ;
#12109=CARTESIAN_POINT ( 'NONE',  ( 8.914835885878215294, 0.000000000000000000, 11.11702303352197418 ) ) ;
#12112=VERTEX_POINT ( 'NONE', #10545 ) ;
#12115=CIRCLE ( 'NONE', #1552, 14.25000000000000178 ) ;
#12118=CARTESIAN_POINT ( 'NONE',  ( 5.733772933379474246, 3.000000000000000000, -13.04554897075799502 ) ) ;
#12120=CARTESIAN_POINT ( 'NONE',  ( -1.557181465540760534, 3.000000000000000000, -14.16466328168009703 ) ) ;
#12130=ORIENTED_EDGE ( 'NONE', *, *, #10550, .T. ) ;
#12132=ADVANCED_FACE ( 'NONE', ( #8199 ), #177, .F. ) ;
#12137=AXIS2_PLACEMENT_3D ( 'NONE', #10914, #5671, #9869 ) ;
#12143=DIRECTION ( 'NONE',  ( 0.000000000000000000, 1.000000000000000000, 0.000000000000000000 ) ) ;
#12150=EDGE_CURVE ( 'NONE', #6731, #1406, #6203, .T. ) ;
#12158=CARTESIAN_POINT ( 'NONE',  ( -8.771102293099080072, 3.000000000000000000, -10.33484986938307770 ) ) ;
#12170=ORIENTED_EDGE ( 'NONE', *, *, #6168, .T. ) ;
#12173=EDGE_CURVE ( 'NONE', #5132, #116, #12499, .T. ) ;
#12175=CARTESIAN_POINT ( 'NONE',  ( 5.797378255456016483, 0.000000000000000000, 12.25282671965375592 ) ) ;
#12183=DIRECTION ( 'NONE',  ( 0.000000000000000000, 0.000000000000000000, -1.000000000000000000 ) ) ;
#12189=ORIENTED_EDGE ( 'NONE', *, *, #5934, .T. ) ;
#12190=AXIS2_PLACEMENT_3D ( 'NONE', #2683, #9480, #6312 ) ;
#12191=CARTESIAN_POINT ( 'NONE',  ( -2.604399508763951321, 0.000000000000000000, 11.80615107470197422 ) ) ;
#12192=AXIS2_PLACEMENT_3D ( 'NONE', #4090, #35, #9246 ) ;
#12202=EDGE_LOOP ( 'NONE', ( #5103, #11468, #7829, #2647 ) ) ;
#12203=CARTESIAN_POINT ( 'NONE',  ( -5.797378255456022700, 0.000000000000000000, -12.25282671965375592 ) ) ;
#12206=CARTESIAN_POINT ( 'NONE',  ( -2.161962830978702677, 3.000000000000000000, 14.08504230442587435 ) ) ;
#12214=CARTESIAN_POINT ( 'NONE',  ( 0.5400000000008007284, 3.000000000000000000, 12.07793442604883793 ) ) ;
#12221=AXIS2_PLACEMENT_3D ( 'NONE', #6568, #7472, #2230 ) ;
#12225=CARTESIAN_POINT ( 'NONE',  ( -0.7702044561450404059, 3.000000000000000000, 12.79759916868914793 ) ) ;
#12226=B_SPLINE_CURVE_WITH_KNOTS ( 'NONE', 3,
 ( #12191, #1715, #673, #4868 ),
 .UNSPECIFIED., .F., .F.,
 ( 4, 4 ),
 ( 0.1547128134717859205, 1.000000000000000000 ),
 .UNSPECIFIED. ) ;
#12229=AXIS2_PLACEMENT_3D ( 'NONE', #1725, #9905, #5913 ) ;
#12235=DIRECTION ( 'NONE',  ( 0.000000000000000000, 1.000000000000000000, 0.000000000000000000 ) ) ;
#12236=ADVANCED_FACE ( 'NONE', ( #409 ), #6609, .T. ) ;
#12240=CARTESIAN_POINT ( 'NONE',  ( 11.48836750521724070, 3.000000000000000000, -8.430890348300621895 ) ) ;
#12241=DIRECTION ( 'NONE',  ( 0.000000000000000000, 1.000000000000000000, 0.000000000000000000 ) ) ;
#12244=ADVANCED_FACE ( 'NONE', ( #7707 ), #10806, .T. ) ;
#12247=ORIENTED_EDGE ( 'NONE', *, *, #10238, .T. ) ;
#12248=ORIENTED_EDGE ( 'NONE', *, *, #7501, .F. ) ;
#12251=B_SPLINE_SURFACE_WITH_KNOTS ( 'NONE', 3, 1, ( 
 ( #1021, #9415 ),
 ( #12282, #11096 ),
 ( #1735, #2822 ),
 ( #4244, #10059 ) ),
 .UNSPECIFIED., .F., .F., .F.,
 ( 4, 4 ),
 ( 2, 2 ),
 ( 0.000000000000000000, 0.8452273900860258760 ),
 ( 0.000000000000000000, 1.000000000000000000 ),
 .UNSPECIFIED. ) ;
#12255=CARTESIAN_POINT ( 'NONE',  ( -5.733772933379540859, 0.000000000000000000, -13.04554897075796660 ) ) ;
#12257=DIRECTION ( 'NONE',  ( -0.000000000000000000, -1.000000000000000000, -0.000000000000000000 ) ) ;
#12269=CARTESIAN_POINT ( 'NONE',  ( 0.000000000000000000, 0.000000000000000000, 0.000000000000000000 ) ) ;
#12275=ORIENTED_EDGE ( 'NONE', *, *, #5373, .F. ) ;
#12282=CARTESIAN_POINT ( 'NONE',  ( -11.14709020439930676, 3.000000000000000000, -7.712570079660886257 ) ) ;
#12286=CARTESIAN_POINT ( 'NONE',  ( -7.712570079660889810, 0.000000000000000000, 11.14709020439930320 ) ) ;
#12287=DIRECTION ( 'NONE',  ( 0.000000000000000000, 1.000000000000000000, 0.000000000000000000 ) ) ;
#12294=ORIENTED_EDGE ( 'NONE', *, *, #3387, .F. ) ;
#12298=CARTESIAN_POINT ( 'NONE',  ( 8.914835885878279242, 3.000000000000000000, 11.11702303352191734 ) ) ;
#12299=CARTESIAN_POINT ( 'NONE',  ( 10.33484986938308481, 3.000000000000000000, -8.771102293099065861 ) ) ;
#12310=B_SPLINE_CURVE_WITH_KNOTS ( 'NONE', 3,
 ( #1104, #216, #4405, #5572 ),
 .UNSPECIFIED., .F., .F.,
 ( 4, 4 ),
 ( 0.000000000000000000, 0.8452273900860258760 ),
 .UNSPECIFIED. ) ;
#12312=ADVANCED_FACE ( 'NONE', ( #7508 ), #2345, .T. ) ;
#12314=CARTESIAN_POINT ( 'NONE',  ( 31.00000000000000000, 3.000000000000000000, -4.000000001073670930 ) ) ;
#12337=LINE ( 'NONE', #12731, #10443 ) ;
#12340=ORIENTED_EDGE ( 'NONE', *, *, #7660, .F. ) ;
#12342=CIRCLE ( 'NONE', #239, 4.000000000000000000 ) ;
#12348=EDGE_CURVE ( 'NONE', #8060, #7270, #12370, .T. ) ;
#12352=CYLINDRICAL_SURFACE ( 'NONE', #10837, 14.25000000000000178 ) ;
#12356=DIRECTION ( 'NONE',  ( 0.000000000000000000, 0.000000000000000000, 1.000000000000000000 ) ) ;
#12358=DIRECTION ( 'NONE',  ( -0.000000000000000000, -1.000000000000000000, -0.000000000000000000 ) ) ;
#12366=ADVANCED_FACE ( 'NONE', ( #1512 ), #5701, .T. ) ;
#12370=B_SPLINE_CURVE_WITH_KNOTS ( 'NONE', 3,
 ( #13153, #2549, #6958, #2607 ),
 .UNSPECIFIED., .F., .F.,
 ( 4, 4 ),
 ( 0.000000000000000000, 0.8452273900860258760 ),
 .UNSPECIFIED. ) ;
#12372=CARTESIAN_POINT ( 'NONE',  ( 9.593885948927676210, 3.000000000000000000, -8.504652361247169168 ) ) ;
#12374=CARTESIAN_POINT ( 'NONE',  ( 13.27898586450067420, 3.000000000000000000, 5.170206418547648397 ) ) ;
#12375=DIRECTION ( 'NONE',  ( -0.000000000000000000, -1.000000000000000000, -0.000000000000000000 ) ) ;
#12378=CARTESIAN_POINT ( 'NONE',  ( -7.077546079049271910, 3.000000000000000000, -10.67828022838850544 ) ) ;
#12382=ORIENTED_EDGE ( 'NONE', *, *, #13345, .T. ) ;
#12390=CARTESIAN_POINT ( 'NONE',  ( 0.5400000000008001733, 0.000000000000000000, 12.07793442604883616 ) ) ;
#12391=DIRECTION ( 'NONE',  ( 0.000000000000000000, 0.000000000000000000, 1.000000000000000000 ) ) ;
#12392=CARTESIAN_POINT ( 'NONE',  ( 6.506507307819716424, 0.000000000000000000, -10.18987059060247269 ) ) ;
#12398=ORIENTED_EDGE ( 'NONE', *, *, #11874, .T. ) ;
#12400=FACE_OUTER_BOUND ( 'NONE', #1306, .T. ) ;
#12402=B_SPLINE_CURVE_WITH_KNOTS ( 'NONE', 3,
 ( #11699, #11906, #8784, #3281 ),
 .UNSPECIFIED., .F., .F.,
 ( 4, 4 ),
 ( 0.000000000000000000, 0.8452273900860258760 ),
 .UNSPECIFIED. ) ;
#12409=CARTESIAN_POINT ( 'NONE',  ( -13.33788847341978645, 0.000000000000000000, -2.414978278956336322 ) ) ;
#12410=CARTESIAN_POINT ( 'NONE',  ( 2.161962830978694683, 3.000000000000000000, -14.08504230442587790 ) ) ;
#12417=CARTESIAN_POINT ( 'NONE',  ( -0.5398653231797316820, 0.000000000000000000, 12.07794044664754018 ) ) ;
#12420=VERTEX_POINT ( 'NONE', #8870 ) ;
#12442=ORIENTED_EDGE ( 'NONE', *, *, #7752, .F. ) ;
#12444=DIRECTION ( 'NONE',  ( -0.000000000000000000, -1.000000000000000000, -0.000000000000000000 ) ) ;
#12447=DIRECTION ( 'NONE',  ( -0.000000000000000000, -1.000000000000000000, -0.000000000000000000 ) ) ;
#12457=LINE ( 'NONE', #6358, #11055 ) ;
#12458=EDGE_LOOP ( 'NONE', ( #3118, #8780, #11172, #9664 ) ) ;
#12464=ORIENTED_EDGE ( 'NONE', *, *, #8643, .T. ) ;
#12472=EDGE_LOOP ( 'NONE', ( #3280, #10851, #11134, #4790 ) ) ;
#12477=EDGE_CURVE ( 'NONE', #3444, #10793, #8552, .T. ) ;
#12478=CARTESIAN_POINT ( 'NONE',  ( 11.46847481510586775, 0.000000000000000000, 5.708888906988908829 ) ) ;
#12480=CARTESIAN_POINT ( 'NONE',  ( -13.33788847341978645, 3.000000000000000000, -2.414978278956336322 ) ) ;
#12481=CARTESIAN_POINT ( 'NONE',  ( 2.161962830978782613, 3.000000000000000000, 14.08504230442586369 ) ) ;
#12482=FACE_OUTER_BOUND ( 'NONE', #5127, .T. ) ;
#12484=CARTESIAN_POINT ( 'NONE',  ( 2.161962830978694683, 0.000000000000000000, -14.08504230442587790 ) ) ;
#12488=ORIENTED_EDGE ( 'NONE', *, *, #12150, .F. ) ;
#12499=LINE ( 'NONE', #7244, #3199 ) ;
#12504=CARTESIAN_POINT ( 'NONE',  ( -11.80612203322752585, 3.000000000000000000, 2.604531154829235362 ) ) ;
#12505=ORIENTED_EDGE ( 'NONE', *, *, #8085, .F. ) ;
#12512=CARTESIAN_POINT ( 'NONE',  ( -13.27898586450066709, 3.000000000000000000, 5.170206418547661720 ) ) ;
#12515=LINE ( 'NONE', #10563, #1874 ) ;
#12516=EDGE_LOOP ( 'NONE', ( #2982, #8225, #8224, #3541 ) ) ;
#12517=CYLINDRICAL_SURFACE ( 'NONE', #11946, 14.25000000000000000 ) ;
#12519=ORIENTED_EDGE ( 'NONE', *, *, #4675, .T. ) ;
#12525=CARTESIAN_POINT ( 'NONE',  ( -14.16466328168009881, 3.000000000000000000, 1.557181465540760534 ) ) ;
#12530=ORIENTED_EDGE ( 'NONE', *, *, #8912, .F. ) ;
#12532=FACE_OUTER_BOUND ( 'NONE', #3843, .T. ) ;
#12541=CARTESIAN_POINT ( 'NONE',  ( -10.34346111134701118, 0.000000000000000000, -8.760376775873707444 ) ) ;
#12545=DIRECTION ( 'NONE',  ( 0.000000000000000000, 0.000000000000000000, 1.000000000000000000 ) ) ;
#12546=CIRCLE ( 'NONE', #2183, 14.25000000000000178 ) ;
#12554=CIRCLE ( 'NONE', #3076, 12.08999999999737440 ) ;
#12556=ORIENTED_EDGE ( 'NONE', *, *, #12477, .F. ) ;
#12558=ORIENTED_EDGE ( 'NONE', *, *, #11390, .F. ) ;
#12559=EDGE_CURVE ( 'NONE', #11264, #8366, #8051, .T. ) ;
#12563=AXIS2_PLACEMENT_3D ( 'NONE', #3737, #6918, #9041 ) ;
#12566=CARTESIAN_POINT ( 'NONE',  ( -5.797378255456022700, 0.000000000000000000, -12.25282671965375592 ) ) ;
#12579=ORIENTED_EDGE ( 'NONE', *, *, #11874, .F. ) ;
#12582=ORIENTED_EDGE ( 'NONE', *, *, #8846, .F. ) ;
#12590=VERTEX_POINT ( 'NONE', #3418 ) ;
#12592=ORIENTED_EDGE ( 'NONE', *, *, #3005, .T. ) ;
#12594=DIRECTION ( 'NONE',  ( 0.000000000000000000, 0.000000000000000000, -1.000000000000000000 ) ) ;
#12598=CLOSED_SHELL ( 'NONE', ( #4109, #3936, #367, #5676, #11245, #12312, #7831, #12244, #8601, #6926, #5236, #2869, #9085, #3212, #8738, #1298, #1583, #433, #12132, #5470, #5756, #4896, #4479, #8519, #12841, #12366, #10767, #10220, #9204, #11593, #9866, #7430, #3484, #2566, #4982, #9890, #11386, #59, #1911, #7679, #878, #3455, #5589, #4389, #7465, #9708, #5742, #10956, #9025, #12797, #3959, #7607, #5981, #10960, #8778, #10867, #1891, #7374, #12977, #7436, #2453, #7029, #153, #13237, #10321, #11834, #1365, #7873, #5936, #7846, #3697, #11811, #11617, #5392, #7935, #13065, #1518, #12724, #13437, #13011, #7454, #917, #6377, #1603, #4114, #8582, #13365, #12236, #10644, #6737, #4397, #957, #11978, #3379, #3279, #3359, #7941 ) ) ;
#12599=CIRCLE ( 'NONE', #11501, 12.08999999999737440 ) ;
#12600=CIRCLE ( 'NONE', #69, 12.08999999999737263 ) ;
#12602=CARTESIAN_POINT ( 'NONE',  ( 5.733772933379453818, 0.000000000000000000, 13.04554897075800568 ) ) ;
#12609=ORIENTED_EDGE ( 'NONE', *, *, #10779, .T. ) ;
#12610=CARTESIAN_POINT ( 'NONE',  ( 0.000000000000000000, 3.000000000000000000, 0.000000000000000000 ) ) ;
#12615=CARTESIAN_POINT ( 'NONE',  ( -11.52662650599083882, 0.000000000000000000, 3.647599401157695986 ) ) ;
#12620=AXIS2_PLACEMENT_3D ( 'NONE', #478, #3775, #10051 ) ;
#12631=AXIS2_PLACEMENT_3D ( 'NONE', #10511, #11550, #9467 ) ;
#12632=CARTESIAN_POINT ( 'NONE',  ( -11.80615107470192804, 0.000000000000000000, -2.604399508764160487 ) ) ;
#12638=CARTESIAN_POINT ( 'NONE',  ( -5.571313494980134173, 0.000000000000000000, 10.72979803820131295 ) ) ;
#12640=CARTESIAN_POINT ( 'NONE',  ( -2.161962830978702677, 3.000000000000000000, 14.08504230442587435 ) ) ;
#12641=ORIENTED_EDGE ( 'NONE', *, *, #4536, .T. ) ;
#12643=CARTESIAN_POINT ( 'NONE',  ( 11.46814821560793618, 0.000000000000000000, -5.731782959214992701 ) ) ;
#12646=ORIENTED_EDGE ( 'NONE', *, *, #10197, .T. ) ;
#12654=CARTESIAN_POINT ( 'NONE',  ( -11.48836750521723893, 3.000000000000000000, 8.430890348300625448 ) ) ;
#12661=VECTOR ( 'NONE', #5034, 1000.000000000000000 ) ;
#12671=CARTESIAN_POINT ( 'NONE',  ( 13.27898586450069907, 0.000000000000000000, 5.170206418547587113 ) ) ;
#12678=ORIENTED_EDGE ( 'NONE', *, *, #6864, .T. ) ;
#12682=DIRECTION ( 'NONE',  ( -0.000000000000000000, -1.000000000000000000, -0.000000000000000000 ) ) ;
#12686=( NAMED_UNIT ( * ) PLANE_ANGLE_UNIT ( ) SI_UNIT ( $, .RADIAN. ) );
#12687=CARTESIAN_POINT ( 'NONE',  ( -12.14623037080100865, 3.000000000000000000, 4.072642252455982437 ) ) ;
#12689=CYLINDRICAL_SURFACE ( 'NONE', #7776, 12.08999999999737440 ) ;
#12693=CARTESIAN_POINT ( 'NONE',  ( -3.647599401157625376, 0.000000000000000000, -11.52662650599085836 ) ) ;
#12697=VERTEX_POINT ( 'NONE', #12108 ) ;
#12703=FACE_OUTER_BOUND ( 'NONE', #11770, .T. ) ;
#12708=DIRECTION ( 'NONE',  ( 0.000000000000000000, 0.000000000000000000, 1.000000000000000000 ) ) ;
#12711=ORIENTED_EDGE ( 'NONE', *, *, #5648, .F. ) ;
#12713=ORIENTED_EDGE ( 'NONE', *, *, #3956, .T. ) ;
#12718=CARTESIAN_POINT ( 'NONE',  ( -4.056222772158361245, 3.000000000000000000, 12.16218796965919324 ) ) ;
#12724=ADVANCED_FACE ( 'NONE', ( #13200 ), #2657, .T. ) ;
#12730=FACE_OUTER_BOUND ( 'NONE', #7840, .T. ) ;
#12731=CARTESIAN_POINT ( 'NONE',  ( -11.52662650599092409, 3.000000000000000000, 3.647599401157420651 ) ) ;
#12736=ORIENTED_EDGE ( 'NONE', *, *, #5607, .T. ) ;
#12740=ORIENTED_EDGE ( 'NONE', *, *, #3807, .F. ) ;
#12744=DIRECTION ( 'NONE',  ( -0.000000000000000000, -1.000000000000000000, -0.000000000000000000 ) ) ;
#12750=( LENGTH_UNIT ( ) NAMED_UNIT ( * ) SI_UNIT ( .MILLI., .METRE. ) );
#12751=EDGE_LOOP ( 'NONE', ( #3012, #10085, #1144, #10687 ) ) ;
#12752=ORIENTED_EDGE ( 'NONE', *, *, #1620, .F. ) ;
#12764=DIRECTION ( 'NONE',  ( 0.000000000000000000, -0.000000000000000000, 1.000000000000000000 ) ) ;
#12766=CARTESIAN_POINT ( 'NONE',  ( 9.593885948927676210, 3.000000000000000000, -8.504652361247169168 ) ) ;
#12767=CARTESIAN_POINT ( 'NONE',  ( 11.48836750521724070, 3.000000000000000000, -8.430890348300621895 ) ) ;
#12768=ORIENTED_EDGE ( 'NONE', *, *, #4056, .F. ) ;
#12770=EDGE_CURVE ( 'NONE', #1091, #11589, #5365, .T. ) ;
#12778=CARTESIAN_POINT ( 'NONE',  ( -0.5398653231797316820, 0.000000000000000000, 12.07794044664754018 ) ) ;
#12782=CARTESIAN_POINT ( 'NONE',  ( 31.00000000000000000, 0.000000000000000000, 3.999999998926329514 ) ) ;
#12784=DIRECTION ( 'NONE',  ( 0.000000000000000000, 0.000000000000000000, -1.000000000000000000 ) ) ;
#12790=AXIS2_PLACEMENT_3D ( 'NONE', #7475, #7544, #8628 ) ;
#12793=CARTESIAN_POINT ( 'NONE',  ( -10.33484986938308303, 0.000000000000000000, 8.771102293099071190 ) ) ;
#12794=CYLINDRICAL_SURFACE ( 'NONE', #8786, 12.08999999999737440 ) ;
#12796=CARTESIAN_POINT ( 'NONE',  ( -12.16218796965919324, 0.000000000000000000, -4.056222772158363021 ) ) ;
#12797=ADVANCED_FACE ( 'NONE', ( #459 ), #4660, .T. ) ;
#12799=AXIS2_PLACEMENT_3D ( 'NONE', #6222, #859, #1058 ) ;
#12806=ORIENTED_EDGE ( 'NONE', *, *, #1541, .T. ) ;
#12807=AXIS2_PLACEMENT_3D ( 'NONE', #11416, #5213, #12594 ) ;
#12808=DIRECTION ( 'NONE',  ( -0.000000000000000000, -1.000000000000000000, -0.000000000000000000 ) ) ;
#12809=B_SPLINE_SURFACE_WITH_KNOTS ( 'NONE', 3, 1, ( 
 ( #5322, #7139 ),
 ( #8221, #4296 ),
 ( #11605, #12643 ),
 ( #1905, #6098 ) ),
 .UNSPECIFIED., .F., .F., .F.,
 ( 4, 4 ),
 ( 2, 2 ),
 ( 0.000000000000000000, 0.8452273900860258760 ),
 ( 0.000000000000000000, 1.000000000000000000 ),
 .UNSPECIFIED. ) ;
#12811=CARTESIAN_POINT ( 'NONE',  ( -11.80612203322752585, 0.000000000000000000, 2.604531154829235362 ) ) ;
#12814=DIRECTION ( 'NONE',  ( -0.000000000000000000, -1.000000000000000000, -0.000000000000000000 ) ) ;
#12821=AXIS2_PLACEMENT_3D ( 'NONE', #10495, #3185, #7394 ) ;
#12827=ORIENTED_EDGE ( 'NONE', *, *, #6084, .T. ) ;
#12828=LINE ( 'NONE', #3380, #7365 ) ;
#12833=EDGE_CURVE ( 'NONE', #1887, #10439, #4939, .T. ) ;
#12839=ORIENTED_EDGE ( 'NONE', *, *, #7746, .F. ) ;
#12841=ADVANCED_FACE ( 'NONE', ( #11413 ), #11705, .F. ) ;
#12843=VECTOR ( 'NONE', #734, 1000.000000000000000 ) ;
#12844=ORIENTED_EDGE ( 'NONE', *, *, #7272, .T. ) ;
#12845=VECTOR ( 'NONE', #11046, 1000.000000000000000 ) ;
#12858=ORIENTED_EDGE ( 'NONE', *, *, #113, .F. ) ;
#12859=VERTEX_POINT ( 'NONE', #13482 ) ;
#12873=AXIS2_PLACEMENT_3D ( 'NONE', #1252, #3244, #6554 ) ;
#12877=B_SPLINE_CURVE_WITH_KNOTS ( 'NONE', 3,
 ( #9828, #8656, #9695, #7496 ),
 .UNSPECIFIED., .F., .F.,
 ( 4, 4 ),
 ( 0.1547128134717859205, 1.000000000000000000 ),
 .UNSPECIFIED. ) ;
#12885=DIRECTION ( 'NONE',  ( 0.000000000000000000, 0.000000000000000000, 1.000000000000000000 ) ) ;
#12892=ORIENTED_EDGE ( 'NONE', *, *, #9144, .F. ) ;
#12894=ORIENTED_EDGE ( 'NONE', *, *, #5264, .F. ) ;
#12898=ORIENTED_EDGE ( 'NONE', *, *, #13410, .T. ) ;
#12902=EDGE_CURVE ( 'NONE', #12046, #8060, #9583, .T. ) ;
#12904=CARTESIAN_POINT ( 'NONE',  ( 0.000000000000000000, 3.000000000000000000, 0.000000000000000000 ) ) ;
#12905=LINE ( 'NONE', #2421, #8867 ) ;
#12906=CARTESIAN_POINT ( 'NONE',  ( -9.593885948927676210, 3.000000000000000000, 8.504652361247165615 ) ) ;
#12907=DIRECTION ( 'NONE',  ( 0.000000000000000000, 1.000000000000000000, 0.000000000000000000 ) ) ;
#12915=LINE ( 'NONE', #12974, #334 ) ;
#12919=CARTESIAN_POINT ( 'NONE',  ( -11.13895890373326836, 0.000000000000000000, 7.723663868796768028 ) ) ;
#12929=CARTESIAN_POINT ( 'NONE',  ( 7.723663868796767140, 3.000000000000000000, 11.13895890373327191 ) ) ;
#12931=CARTESIAN_POINT ( 'NONE',  ( 8.158551673544282679, 3.000000000000000000, -8.922226997226884393 ) ) ;
#12935=CARTESIAN_POINT ( 'NONE',  ( 12.46219022525837694, 0.000000000000000000, -4.344528055836598845 ) ) ;
#12936=VERTEX_POINT ( 'NONE', #12100 ) ;
#12937=ORIENTED_EDGE ( 'NONE', *, *, #8613, .F. ) ;
#12941=DIRECTION ( 'NONE',  ( 0.000000000000000000, 0.000000000000000000, 1.000000000000000000 ) ) ;
#12943=CARTESIAN_POINT ( 'NONE',  ( 5.708888906988906164, 0.000000000000000000, -11.46847481510586775 ) ) ;
#12944=LINE ( 'NONE', #8996, #2652 ) ;
#12947=FACE_OUTER_BOUND ( 'NONE', #3797, .T. ) ;
#12948=DIRECTION ( 'NONE',  ( -0.000000000000000000, -1.000000000000000000, -0.000000000000000000 ) ) ;
#12958=DIRECTION ( 'NONE',  ( 0.000000000000000000, 0.000000000000000000, 1.000000000000000000 ) ) ;
#12968=CARTESIAN_POINT ( 'NONE',  ( 0.000000000000000000, 0.000000000000000000, 0.000000000000000000 ) ) ;
#12970=ORIENTED_EDGE ( 'NONE', *, *, #3064, .T. ) ;
#12974=CARTESIAN_POINT ( 'NONE',  ( -14.08504230442587790, 3.000000000000000000, -2.161962830978695571 ) ) ;
#12975=CARTESIAN_POINT ( 'NONE',  ( 11.14709020439929787, 3.000000000000000000, 7.712570079660892475 ) ) ;
#12977=ADVANCED_FACE ( 'NONE', ( #8772 ), #6540, .F. ) ;
#12991=CIRCLE ( 'NONE', #1114, 14.24999999999999822 ) ;
#12996=CARTESIAN_POINT ( 'NONE',  ( -0.7901945867173586491, 3.000000000000000000, -12.78643498603818074 ) ) ;
#13004=ORIENTED_EDGE ( 'NONE', *, *, #12015, .F. ) ;
#13006=CARTESIAN_POINT ( 'NONE',  ( 8.922226997226882617, 0.000000000000000000, 8.158551673544282679 ) ) ;
#13008=CARTESIAN_POINT ( 'NONE',  ( 5.571313494980132397, 0.000000000000000000, -10.72979803820131472 ) ) ;
#13011=ADVANCED_FACE ( 'NONE', ( #13062 ), #3618, .T. ) ;
#13013=CARTESIAN_POINT ( 'NONE',  ( 5.708888906988906164, 3.000000000000000000, -11.46847481510586775 ) ) ;
#13022=DIRECTION ( 'NONE',  ( -0.000000000000000000, -1.000000000000000000, -0.000000000000000000 ) ) ;
#13029=VECTOR ( 'NONE', #2611, 1000.000000000000000 ) ;
#13038=ORIENTED_EDGE ( 'NONE', *, *, #8339, .T. ) ;
#13039=ORIENTED_EDGE ( 'NONE', *, *, #8254, .F. ) ;
#13040=AXIS2_PLACEMENT_3D ( 'NONE', #1935, #4188, #9372 ) ;
#13042=VECTOR ( 'NONE', #10233, 1000.000000000000000 ) ;
#13047=DIRECTION ( 'NONE',  ( 0.000000000000000000, 0.000000000000000000, 1.000000000000000000 ) ) ;
#13054=CIRCLE ( 'NONE', #11728, 1.499999999686092877 ) ;
#13055=ORIENTED_EDGE ( 'NONE', *, *, #6999, .T. ) ;
#13062=FACE_OUTER_BOUND ( 'NONE', #482, .T. ) ;
#13065=ADVANCED_FACE ( 'NONE', ( #9051 ), #5136, .T. ) ;
#13072=AXIS2_PLACEMENT_3D ( 'NONE', #13363, #8115, #10466 ) ;
#13079=EDGE_CURVE ( 'NONE', #13528, #11718, #1412, .T. ) ;
#13085=DIRECTION ( 'NONE',  ( 0.000000000000000000, 0.000000000000000000, 1.000000000000000000 ) ) ;
#13087=CARTESIAN_POINT ( 'NONE',  ( -5.733772933379540859, 3.000000000000000000, -13.04554897075796660 ) ) ;
#13090=ORIENTED_EDGE ( 'NONE', *, *, #3550, .T. ) ;
#13108=CARTESIAN_POINT ( 'NONE',  ( 3.647599401157688437, 3.000000000000000000, 11.52662650599083882 ) ) ;
#13109=ORIENTED_EDGE ( 'NONE', *, *, #6647, .F. ) ;
#13111=EDGE_LOOP ( 'NONE', ( #4553, #625, #8400, #12609 ) ) ;
#13112=PRODUCT_DEFINITION_FORMATION_WITH_SPECIFIED_SOURCE ( 'ANY', '', #8958, .NOT_KNOWN. ) ;
#13125=EDGE_CURVE ( 'NONE', #9840, #12067, #3891, .T. ) ;
#13127=VERTEX_POINT ( 'NONE', #7148 ) ;
#13128=CARTESIAN_POINT ( 'NONE',  ( 5.733772933379541747, 3.000000000000000000, 13.04554897075796482 ) ) ;
#13131=DIRECTION ( 'NONE',  ( -0.000000000000000000, -1.000000000000000000, -0.000000000000000000 ) ) ;
#13132=DIRECTION ( 'NONE',  ( -0.000000000000000000, -1.000000000000000000, -0.000000000000000000 ) ) ;
#13134=EDGE_CURVE ( 'NONE', #11941, #9276, #6048, .T. ) ;
#13137=CARTESIAN_POINT ( 'NONE',  ( 12.01285915242476499, 0.000000000000000000, -4.000000001073668265 ) ) ;
#13138=VERTEX_POINT ( 'NONE', #12525 ) ;
#13148=CARTESIAN_POINT ( 'NONE',  ( 0.000000000000000000, 0.000000000000000000, 0.000000000000000000 ) ) ;
#13149=B_SPLINE_CURVE_WITH_KNOTS ( 'NONE', 3,
 ( #10829, #233, #10636, #1259 ),
 .UNSPECIFIED., .F., .F.,
 ( 4, 4 ),
 ( 0.1547128134717859205, 1.000000000000000000 ),
 .UNSPECIFIED. ) ;
#13150=DIRECTION ( 'NONE',  ( -0.000000000000000000, -1.000000000000000000, -0.000000000000000000 ) ) ;
#13153=CARTESIAN_POINT ( 'NONE',  ( 2.161962830978677363, 0.000000000000000000, 14.08504230442587613 ) ) ;
#13160=CARTESIAN_POINT ( 'NONE',  ( -7.712570079660889810, 3.000000000000000000, 11.14709020439930320 ) ) ;
#13163=ORIENTED_EDGE ( 'NONE', *, *, #8503, .T. ) ;
#13168=CARTESIAN_POINT ( 'NONE',  ( -5.571433138827826426, 0.000000000000000000, -10.72973591378220526 ) ) ;
#13174=ORIENTED_EDGE ( 'NONE', *, *, #1620, .T. ) ;
#13177=CARTESIAN_POINT ( 'NONE',  ( 4.564691384634508964, 3.000000000000000000, -12.76342233970727413 ) ) ;
#13178=CARTESIAN_POINT ( 'NONE',  ( 5.170206418547604876, 3.000000000000000000, -13.27898586450069196 ) ) ;
#13179=CARTESIAN_POINT ( 'NONE',  ( -10.72973591378220348, 3.000000000000000000, 5.571433138827830867 ) ) ;
#13181=CARTESIAN_POINT ( 'NONE',  ( -8.914835885878282795, 3.000000000000000000, -11.11702303352191556 ) ) ;
#13187=LINE ( 'NONE', #1833, #5768 ) ;
#13188=ORIENTED_EDGE ( 'NONE', *, *, #5333, .T. ) ;
#13195=AXIS2_PLACEMENT_3D ( 'NONE', #4795, #10244, #8981 ) ;
#13196=DIRECTION ( 'NONE',  ( 0.000000000000000000, 0.000000000000000000, -1.000000000000000000 ) ) ;
#13199=DIRECTION ( 'NONE',  ( -0.000000000000000000, -1.000000000000000000, -0.000000000000000000 ) ) ;
#13200=FACE_OUTER_BOUND ( 'NONE', #2228, .T. ) ;
#13202=ORIENTED_EDGE ( 'NONE', *, *, #5648, .T. ) ;
#13212=LINE ( 'NONE', #1371, #2440 ) ;
#13214=PLANE ( 'NONE',  #115 ) ;
#13220=CARTESIAN_POINT ( 'NONE',  ( -5.733772933379541747, 3.000000000000000000, -13.04554897075796482 ) ) ;
#13225=LINE ( 'NONE', #5921, #8208 ) ;
#13226=VECTOR ( 'NONE', #5949, 1000.000000000000000 ) ;
#13234=CARTESIAN_POINT ( 'NONE',  ( 1.557181465540758758, 0.000000000000000000, 14.16466328168009881 ) ) ;
#13236=CARTESIAN_POINT ( 'NONE',  ( 11.48836750521724070, 0.000000000000000000, 8.430890348300627224 ) ) ;
#13237=ADVANCED_FACE ( 'NONE', ( #8494 ), #3257, .T. ) ;
#13240=ORIENTED_EDGE ( 'NONE', *, *, #4313, .T. ) ;
#13244=VERTEX_POINT ( 'NONE', #9605 ) ;
#13246=B_SPLINE_CURVE_WITH_KNOTS ( 'NONE', 3,
 ( #10393, #5090, #5023, #12484 ),
 .UNSPECIFIED., .F., .F.,
 ( 4, 4 ),
 ( 0.1547128134717859205, 1.000000000000000000 ),
 .UNSPECIFIED. ) ;
#13248=EDGE_CURVE ( 'NONE', #2012, #8754, #985, .T. ) ;
#13251=CARTESIAN_POINT ( 'NONE',  ( 11.11702303352191912, 0.000000000000000000, -8.914835885878277466 ) ) ;
#13262=ORIENTED_EDGE ( 'NONE', *, *, #2334, .T. ) ;
#13265=AXIS2_PLACEMENT_3D ( 'NONE', #6922, #4992, #11050 ) ;
#13268=VERTEX_POINT ( 'NONE', #8818 ) ;
#13279=CARTESIAN_POINT ( 'NONE',  ( -0.5398653231797316820, 0.000000000000000000, 12.07794044664754018 ) ) ;
#13290=DIRECTION ( 'NONE',  ( 0.000000000000000000, 0.000000000000000000, 1.000000000000000000 ) ) ;
#13292=CARTESIAN_POINT ( 'NONE',  ( 0.000000000000000000, 3.000000000000000000, -12.08999999999737440 ) ) ;
#13293=AXIS2_PLACEMENT_3D ( 'NONE', #2077, #10481, #839 ) ;
#13298=VERTEX_POINT ( 'NONE', #10910 ) ;
#13300=EDGE_CURVE ( 'NONE', #8949, #4662, #7863, .T. ) ;
#13314=DIRECTION ( 'NONE',  ( -0.000000000000000000, -1.000000000000000000, -0.000000000000000000 ) ) ;
#13318=CARTESIAN_POINT ( 'NONE',  ( 4.577511697546072789, 3.000000000000000000, 12.75843939030335505 ) ) ;
#13326=VERTEX_POINT ( 'NONE', #3463 ) ;
#13333=CARTESIAN_POINT ( 'NONE',  ( 10.34346111134700585, 0.000000000000000000, 8.760376775873716326 ) ) ;
#13338=CARTESIAN_POINT ( 'NONE',  ( 11.48836750521724070, 0.000000000000000000, -8.430890348300621895 ) ) ;
#13340=EDGE_CURVE ( 'NONE', #7698, #8964, #12915, .T. ) ;
#13343=ORIENTED_EDGE ( 'NONE', *, *, #3633, .F. ) ;
#13345=EDGE_CURVE ( 'NONE', #4061, #3444, #9347, .T. ) ;
#13354=CARTESIAN_POINT ( 'NONE',  ( -13.04554897075799680, 0.000000000000000000, -5.733772933379471581 ) ) ;
#13357=CARTESIAN_POINT ( 'NONE',  ( 0.000000000000000000, 3.000000000000000000, 0.000000000000000000 ) ) ;
#13359=CARTESIAN_POINT ( 'NONE',  ( 0.000000000000000000, 3.000000000000000000, 0.000000000000000000 ) ) ;
#13361=DIRECTION ( 'NONE',  ( 0.000000000000000000, 0.000000000000000000, -1.000000000000000000 ) ) ;
#13363=CARTESIAN_POINT ( 'NONE',  ( 0.000000000000000000, 3.000000000000000000, 0.000000000000000000 ) ) ;
#13365=ADVANCED_FACE ( 'NONE', ( #379 ), #8502, .F. ) ;
#13367=EDGE_CURVE ( 'NONE', #10549, #2066, #2930, .T. ) ;
#13369=FACE_OUTER_BOUND ( 'NONE', #4108, .T. ) ;
#13373=ORIENTED_EDGE ( 'NONE', *, *, #12902, .F. ) ;
#13379=LINE ( 'NONE', #7183, #972 ) ;
#13390=CARTESIAN_POINT ( 'NONE',  ( 8.914835885878279242, 0.000000000000000000, 11.11702303352191734 ) ) ;
#13398=LINE ( 'NONE', #11336, #2713 ) ;
#13410=EDGE_CURVE ( 'NONE', #284, #7698, #5074, .T. ) ;
#13413=DIRECTION ( 'NONE',  ( 0.000000000000000000, 1.000000000000000000, 0.000000000000000000 ) ) ;
#13414=FACE_OUTER_BOUND ( 'NONE', #3591, .T. ) ;
#13420=EDGE_CURVE ( 'NONE', #8421, #11907, #4905, .T. ) ;
#13422=CARTESIAN_POINT ( 'NONE',  ( 0.000000000000000000, 3.000000000000000000, 0.000000000000000000 ) ) ;
#13423=CARTESIAN_POINT ( 'NONE',  ( -12.55526518755974585, 3.000000000000000000, -2.546103534247746047 ) ) ;
#13429=CARTESIAN_POINT ( 'NONE',  ( -9.600126836553261711, 3.000000000000000000, -8.482622935103767858 ) ) ;
#13431=ORIENTED_EDGE ( 'NONE', *, *, #9016, .F. ) ;
#13437=ADVANCED_FACE ( 'NONE', ( #9177 ), #3228, .F. ) ;
#13439=CARTESIAN_POINT ( 'NONE',  ( -11.14709020439930676, 0.000000000000000000, -7.712570079660886257 ) ) ;
#13441=VECTOR ( 'NONE', #6418, 1000.000000000000000 ) ;
#13446=EDGE_CURVE ( 'NONE', #7415, #1162, #2777, .T. ) ;
#13449=B_SPLINE_CURVE_WITH_KNOTS ( 'NONE', 3,
 ( #5371, #9578, #7507, #9640 ),
 .UNSPECIFIED., .F., .F.,
 ( 4, 4 ),
 ( 0.000000000000000000, 0.8452273900860258760 ),
 .UNSPECIFIED. ) ;
#13460=DIRECTION ( 'NONE',  ( 0.000000000000000000, 0.000000000000000000, 1.000000000000000000 ) ) ;
#13465=CARTESIAN_POINT ( 'NONE',  ( -7.723663868796776910, 0.000000000000000000, -11.13895890373326303 ) ) ;
#13473=AXIS2_PLACEMENT_3D ( 'NONE', #3261, #11294, #4314 ) ;
#13480=CIRCLE ( 'NONE', #8404, 14.24999999999999822 ) ;
#13482=CARTESIAN_POINT ( 'NONE',  ( 8.430890348300586368, 3.000000000000000000, -11.48836750521726913 ) ) ;
#13483=CARTESIAN_POINT ( 'NONE',  ( -14.08504230442587790, 0.000000000000000000, -2.161962830978695571 ) ) ;
#13490=VECTOR ( 'NONE', #3753, 1000.000000000000000 ) ;
#13495=CARTESIAN_POINT ( 'NONE',  ( 0.5400000000008001733, 3.000000000000000000, 12.07793442604883616 ) ) ;
#13496=CARTESIAN_POINT ( 'NONE',  ( 4.564691384634508964, 0.000000000000000000, -12.76342233970727413 ) ) ;
#13497=CARTESIAN_POINT ( 'NONE',  ( 5.571433138827823761, 0.000000000000000000, 10.72973591378220704 ) ) ;
#13499=B_SPLINE_CURVE_WITH_KNOTS ( 'NONE', 3,
 ( #6524, #8573, #12796, #7559 ),
 .UNSPECIFIED., .F., .F.,
 ( 4, 4 ),
 ( 0.000000000000000000, 0.8452273900860258760 ),
 .UNSPECIFIED. ) ;
#13500=VECTOR ( 'NONE', #11543, 1000.000000000000000 ) ;
#13505=ORIENTED_EDGE ( 'NONE', *, *, #4761, .T. ) ;
#13512=( NAMED_UNIT ( * ) SI_UNIT ( $, .STERADIAN. ) SOLID_ANGLE_UNIT ( ) );
#13528=VERTEX_POINT ( 'NONE', #3308 ) ;
#13530=CARTESIAN_POINT ( 'NONE',  ( 8.922136023539611216, 0.000000000000000000, -8.158651161643899030 ) ) ;
#13531=CARTESIAN_POINT ( 'NONE',  ( 7.723663868796767140, 3.000000000000000000, 11.13895890373327191 ) ) ;
#13532=CARTESIAN_POINT ( 'NONE',  ( -2.604531154829235362, 3.000000000000000000, -11.80612203322752585 ) ) ;
#13533=CARTESIAN_POINT ( 'NONE',  ( 31.00000000000000000, 3.000000000000000000, -1.073670993220974656E-09 ) ) ;
#13535=AXIS2_PLACEMENT_3D ( 'NONE', #6898, #6007, #10211 ) ;
#13538=CARTESIAN_POINT ( 'NONE',  ( -7.723663868796776910, 0.000000000000000000, -11.13895890373326303 ) ) ;
#13540=ORIENTED_EDGE ( 'NONE', *, *, #5835, .F. ) ;
#13548=DIRECTION ( 'NONE',  ( -0.000000000000000000, -1.000000000000000000, -0.000000000000000000 ) ) ;
#13552=CARTESIAN_POINT ( 'NONE',  ( -14.16466328168010769, 0.000000000000000000, -1.557181465540670384 ) ) ;
#13553=CARTESIAN_POINT ( 'NONE',  ( -1.557181465540677712, 3.000000000000000000, 14.16466328168010769 ) ) ;
#13556=DIRECTION ( 'NONE',  ( -0.000000000000000000, -1.000000000000000000, -0.000000000000000000 ) ) ;
#13559=CYLINDRICAL_SURFACE ( 'NONE', #3152, 12.08999999999737440 ) ;
#13562=DIRECTION ( 'NONE',  ( 0.000000000000000000, 0.000000000000000000, 1.000000000000000000 ) ) ;
#13564=EDGE_CURVE ( 'NONE', #4061, #2104, #7520, .T. ) ;
#13568=EDGE_LOOP ( 'NONE', ( #10764, #12530, #1460, #13174 ) ) ;
#13569=ORIENTED_EDGE ( 'NONE', *, *, #4365, .F. ) ;
#13574=CYLINDRICAL_SURFACE ( 'NONE', #8406, 12.08999999999737440 ) ;
#13576=LINE ( 'NONE', #6199, #9018 ) ;
#13578=EDGE_CURVE ( 'NONE', #1090, #8924, #3045, .T. ) ;
#13580=CARTESIAN_POINT ( 'NONE',  ( -13.04554897075799680, 0.000000000000000000, -5.733772933379471581 ) ) ;
#13586=ORIENTED_EDGE ( 'NONE', *, *, #4365, .T. ) ;
#13588=ORIENTED_EDGE ( 'NONE', *, *, #10021, .T. ) ;
#13591=CARTESIAN_POINT ( 'NONE',  ( 2.604399508763944660, 3.000000000000000000, -11.80615107470197600 ) ) ;
#13593=CARTESIAN_POINT ( 'NONE',  ( 9.600126836553261711, 0.000000000000000000, 8.482622935103766082 ) ) ;
#13594=CARTESIAN_POINT ( 'NONE',  ( -5.571313494980132397, 3.000000000000000000, 10.72979803820132005 ) ) ;
#13636=COLOUR_RGB('Sky Blue',0.24,0.69,0.87);
#13637=FILL_AREA_STYLE_COLOUR('',#13636);
#13638=FILL_AREA_STYLE('',(#13637));
#13639=SURFACE_STYLE_FILL_AREA(#13638);
#13640=SURFACE_SIDE_STYLE('',(#13639));
#13641=SURFACE_STYLE_USAGE(.BOTH.,#13640);
#13642=PRESENTATION_STYLE_ASSIGNMENT((#13641));
ENDSEC;
END-ISO-10303-21;
